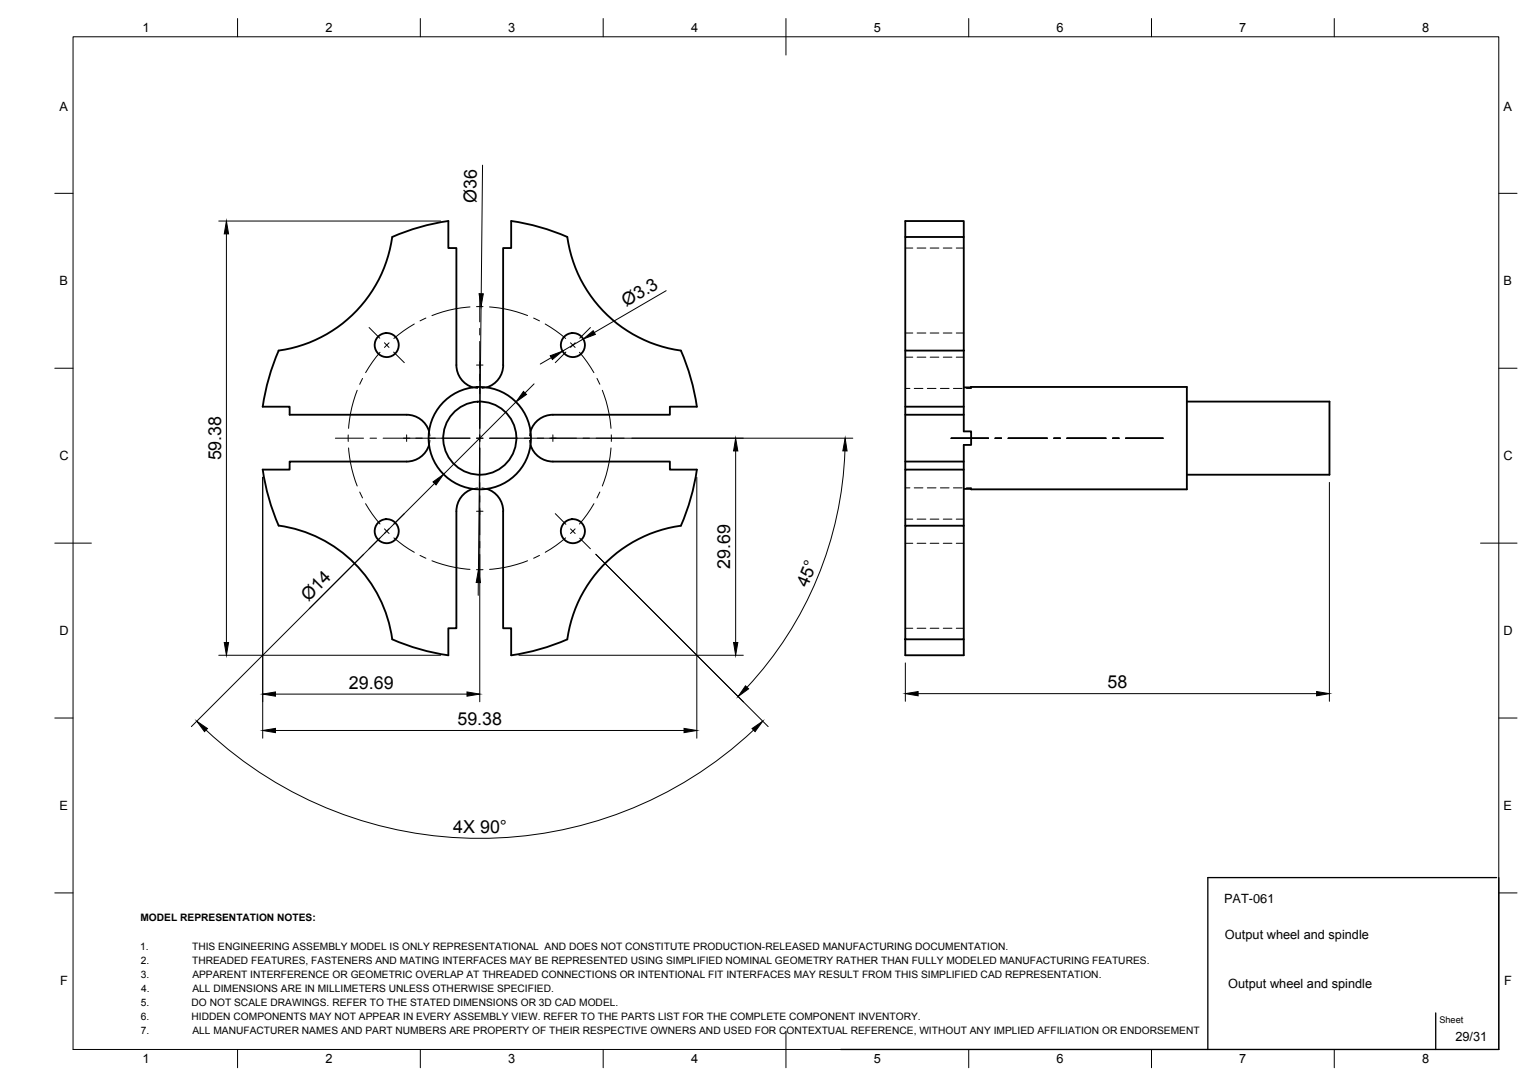
ISO-10303-21;
HEADER;
/* Generated by software containing ST-Developer
 * from STEP Tools, Inc. (www.steptools.com) 
 */

FILE_DESCRIPTION(
/* description */ ('Compact intermittent indexer'),
/* implementation_level */ '2;1');

FILE_NAME(
/* name */ 'Output wheel and spindle.step',
/* time_stamp */ '2026-10-29T16:32:17-07:00',
/* author */ (''),
/* organization */ (''),
/* preprocessor_version */ 'ST-DEVELOPER v20.2',
/* originating_system */ 'Autodesk Translation Framework v15.17.0.0',
/* authorisation */ '');

FILE_SCHEMA (('AUTOMOTIVE_DESIGN { 1 0 10303 214 3 1 1 }'));
ENDSEC;

DATA;
#10=MECHANICAL_DESIGN_GEOMETRIC_PRESENTATION_REPRESENTATION('',(#285),#10837);
#229=SHAPE_REPRESENTATION_RELATIONSHIP('SRR','None',#10966,#253);
#253=ADVANCED_BREP_SHAPE_REPRESENTATION('',(#315),#10833);
#285=STYLED_ITEM('',(#11159),#315);
#315=MANIFOLD_SOLID_BREP('Body1',#5659);
#455=FACE_BOUND('',#1346,.T.);
#456=FACE_BOUND('',#1347,.T.);
#457=FACE_BOUND('',#1348,.T.);
#458=FACE_BOUND('',#1349,.T.);
#459=FACE_BOUND('',#1358,.T.);
#460=FACE_BOUND('',#1360,.T.);
#461=FACE_BOUND('',#1372,.T.);
#462=FACE_BOUND('',#1383,.T.);
#463=FACE_BOUND('',#1397,.T.);
#600=PLANE('',#6521);
#601=PLANE('',#6535);
#602=PLANE('',#6536);
#603=PLANE('',#6537);
#604=PLANE('',#6538);
#605=PLANE('',#6539);
#606=PLANE('',#6540);
#607=PLANE('',#6545);
#608=PLANE('',#6549);
#609=PLANE('',#6561);
#610=PLANE('',#6563);
#611=PLANE('',#6564);
#612=PLANE('',#6565);
#613=PLANE('',#6566);
#614=PLANE('',#6567);
#615=PLANE('',#6568);
#616=PLANE('',#6572);
#617=PLANE('',#6575);
#618=PLANE('',#6577);
#619=PLANE('',#6578);
#620=PLANE('',#6579);
#621=PLANE('',#6580);
#622=PLANE('',#6581);
#623=PLANE('',#6582);
#624=PLANE('',#6586);
#625=PLANE('',#6589);
#626=PLANE('',#6591);
#627=PLANE('',#6592);
#628=PLANE('',#6593);
#629=PLANE('',#6594);
#630=PLANE('',#6595);
#631=PLANE('',#6598);
#632=PLANE('',#6599);
#633=PLANE('',#6600);
#634=PLANE('',#6604);
#904=FACE_OUTER_BOUND('',#1334,.T.);
#905=FACE_OUTER_BOUND('',#1335,.T.);
#906=FACE_OUTER_BOUND('',#1336,.T.);
#907=FACE_OUTER_BOUND('',#1337,.T.);
#908=FACE_OUTER_BOUND('',#1338,.T.);
#909=FACE_OUTER_BOUND('',#1339,.T.);
#910=FACE_OUTER_BOUND('',#1340,.T.);
#911=FACE_OUTER_BOUND('',#1341,.T.);
#912=FACE_OUTER_BOUND('',#1342,.T.);
#913=FACE_OUTER_BOUND('',#1343,.T.);
#914=FACE_OUTER_BOUND('',#1344,.T.);
#915=FACE_OUTER_BOUND('',#1345,.T.);
#916=FACE_OUTER_BOUND('',#1350,.T.);
#917=FACE_OUTER_BOUND('',#1351,.T.);
#918=FACE_OUTER_BOUND('',#1352,.T.);
#919=FACE_OUTER_BOUND('',#1353,.T.);
#920=FACE_OUTER_BOUND('',#1354,.T.);
#921=FACE_OUTER_BOUND('',#1355,.T.);
#922=FACE_OUTER_BOUND('',#1356,.T.);
#923=FACE_OUTER_BOUND('',#1357,.T.);
#924=FACE_OUTER_BOUND('',#1359,.T.);
#925=FACE_OUTER_BOUND('',#1361,.T.);
#926=FACE_OUTER_BOUND('',#1362,.T.);
#927=FACE_OUTER_BOUND('',#1363,.T.);
#928=FACE_OUTER_BOUND('',#1364,.T.);
#929=FACE_OUTER_BOUND('',#1365,.T.);
#930=FACE_OUTER_BOUND('',#1366,.T.);
#931=FACE_OUTER_BOUND('',#1367,.T.);
#932=FACE_OUTER_BOUND('',#1368,.T.);
#933=FACE_OUTER_BOUND('',#1369,.T.);
#934=FACE_OUTER_BOUND('',#1370,.T.);
#935=FACE_OUTER_BOUND('',#1371,.T.);
#936=FACE_OUTER_BOUND('',#1373,.T.);
#937=FACE_OUTER_BOUND('',#1374,.T.);
#938=FACE_OUTER_BOUND('',#1375,.T.);
#939=FACE_OUTER_BOUND('',#1376,.T.);
#940=FACE_OUTER_BOUND('',#1377,.T.);
#941=FACE_OUTER_BOUND('',#1378,.T.);
#942=FACE_OUTER_BOUND('',#1379,.T.);
#943=FACE_OUTER_BOUND('',#1380,.T.);
#944=FACE_OUTER_BOUND('',#1381,.T.);
#945=FACE_OUTER_BOUND('',#1382,.T.);
#946=FACE_OUTER_BOUND('',#1384,.T.);
#947=FACE_OUTER_BOUND('',#1385,.T.);
#948=FACE_OUTER_BOUND('',#1386,.T.);
#949=FACE_OUTER_BOUND('',#1387,.T.);
#950=FACE_OUTER_BOUND('',#1388,.T.);
#951=FACE_OUTER_BOUND('',#1389,.T.);
#952=FACE_OUTER_BOUND('',#1390,.T.);
#953=FACE_OUTER_BOUND('',#1391,.T.);
#954=FACE_OUTER_BOUND('',#1392,.T.);
#955=FACE_OUTER_BOUND('',#1393,.T.);
#956=FACE_OUTER_BOUND('',#1394,.T.);
#957=FACE_OUTER_BOUND('',#1395,.T.);
#958=FACE_OUTER_BOUND('',#1396,.T.);
#959=FACE_OUTER_BOUND('',#1398,.T.);
#960=FACE_OUTER_BOUND('',#1399,.T.);
#1334=EDGE_LOOP('',(#4732,#4733,#4734,#4735));
#1335=EDGE_LOOP('',(#4736,#4737,#4738,#4739));
#1336=EDGE_LOOP('',(#4740,#4741,#4742,#4743));
#1337=EDGE_LOOP('',(#4744,#4745,#4746,#4747));
#1338=EDGE_LOOP('',(#4748,#4749,#4750,#4751));
#1339=EDGE_LOOP('',(#4752,#4753,#4754,#4755));
#1340=EDGE_LOOP('',(#4756,#4757,#4758,#4759));
#1341=EDGE_LOOP('',(#4760,#4761,#4762,#4763));
#1342=EDGE_LOOP('',(#4764,#4765,#4766,#4767));
#1343=EDGE_LOOP('',(#4768,#4769,#4770,#4771));
#1344=EDGE_LOOP('',(#4772,#4773,#4774,#4775));
#1345=EDGE_LOOP('',(#4776,#4777,#4778,#4779,#4780,#4781,#4782,#4783,#4784,
#4785,#4786,#4787,#4788,#4789,#4790,#4791,#4792,#4793,#4794,#4795,#4796,
#4797,#4798,#4799,#4800,#4801,#4802,#4803,#4804,#4805,#4806,#4807,#4808,
#4809,#4810,#4811,#4812,#4813,#4814,#4815));
#1346=EDGE_LOOP('',(#4816));
#1347=EDGE_LOOP('',(#4817));
#1348=EDGE_LOOP('',(#4818));
#1349=EDGE_LOOP('',(#4819));
#1350=EDGE_LOOP('',(#4820,#4821,#4822,#4823));
#1351=EDGE_LOOP('',(#4824,#4825,#4826,#4827));
#1352=EDGE_LOOP('',(#4828,#4829,#4830,#4831));
#1353=EDGE_LOOP('',(#4832,#4833,#4834,#4835));
#1354=EDGE_LOOP('',(#4836,#4837,#4838,#4839));
#1355=EDGE_LOOP('',(#4840,#4841,#4842,#4843));
#1356=EDGE_LOOP('',(#4844,#4845,#4846,#4847));
#1357=EDGE_LOOP('',(#4848,#4849,#4850,#4851,#4852,#4853,#4854,#4855,#4856,
#4857,#4858,#4859));
#1358=EDGE_LOOP('',(#4860));
#1359=EDGE_LOOP('',(#4861,#4862,#4863,#4864,#4865,#4866,#4867,#4868,#4869,
#4870,#4871,#4872));
#1360=EDGE_LOOP('',(#4873));
#1361=EDGE_LOOP('',(#4874,#4875));
#1362=EDGE_LOOP('',(#4876,#4877,#4878,#4879,#4880,#4881,#4882,#4883));
#1363=EDGE_LOOP('',(#4884,#4885,#4886,#4887,#4888,#4889,#4890,#4891,#4892,
#4893,#4894,#4895,#4896,#4897,#4898,#4899,#4900,#4901,#4902,#4903));
#1364=EDGE_LOOP('',(#4904,#4905,#4906,#4907));
#1365=EDGE_LOOP('',(#4908,#4909,#4910,#4911));
#1366=EDGE_LOOP('',(#4912,#4913,#4914,#4915));
#1367=EDGE_LOOP('',(#4916,#4917,#4918,#4919));
#1368=EDGE_LOOP('',(#4920,#4921,#4922,#4923));
#1369=EDGE_LOOP('',(#4924,#4925,#4926,#4927));
#1370=EDGE_LOOP('',(#4928,#4929,#4930,#4931));
#1371=EDGE_LOOP('',(#4932,#4933,#4934,#4935,#4936,#4937,#4938,#4939,#4940,
#4941,#4942,#4943));
#1372=EDGE_LOOP('',(#4944));
#1373=EDGE_LOOP('',(#4945,#4946,#4947));
#1374=EDGE_LOOP('',(#4948,#4949,#4950,#4951,#4952,#4953,#4954,#4955));
#1375=EDGE_LOOP('',(#4956,#4957,#4958,#4959));
#1376=EDGE_LOOP('',(#4960,#4961,#4962,#4963));
#1377=EDGE_LOOP('',(#4964,#4965,#4966,#4967));
#1378=EDGE_LOOP('',(#4968,#4969,#4970,#4971));
#1379=EDGE_LOOP('',(#4972,#4973,#4974,#4975));
#1380=EDGE_LOOP('',(#4976,#4977,#4978,#4979));
#1381=EDGE_LOOP('',(#4980,#4981,#4982,#4983));
#1382=EDGE_LOOP('',(#4984,#4985,#4986,#4987,#4988,#4989,#4990,#4991,#4992,
#4993,#4994,#4995));
#1383=EDGE_LOOP('',(#4996));
#1384=EDGE_LOOP('',(#4997,#4998));
#1385=EDGE_LOOP('',(#4999,#5000,#5001,#5002,#5003,#5004,#5005,#5006));
#1386=EDGE_LOOP('',(#5007,#5008,#5009,#5010));
#1387=EDGE_LOOP('',(#5011,#5012,#5013,#5014));
#1388=EDGE_LOOP('',(#5015,#5016,#5017,#5018));
#1389=EDGE_LOOP('',(#5019,#5020,#5021,#5022));
#1390=EDGE_LOOP('',(#5023,#5024,#5025,#5026));
#1391=EDGE_LOOP('',(#5027,#5028,#5029,#5030));
#1392=EDGE_LOOP('',(#5031,#5032));
#1393=EDGE_LOOP('',(#5033,#5034,#5035,#5036,#5037,#5038,#5039,#5040));
#1394=EDGE_LOOP('',(#5041,#5042,#5043,#5044));
#1395=EDGE_LOOP('',(#5045,#5046,#5047,#5048));
#1396=EDGE_LOOP('',(#5049));
#1397=EDGE_LOOP('',(#5050));
#1398=EDGE_LOOP('',(#5051,#5052,#5053,#5054));
#1399=EDGE_LOOP('',(#5055));
#1656=LINE('',#10192,#2014);
#1657=LINE('',#10198,#2015);
#1658=LINE('',#10204,#2016);
#1659=LINE('',#10210,#2017);
#1660=LINE('',#10217,#2018);
#1661=LINE('',#10220,#2019);
#1662=LINE('',#10226,#2020);
#1663=LINE('',#10229,#2021);
#1664=LINE('',#10235,#2022);
#1665=LINE('',#10238,#2023);
#1666=LINE('',#10242,#2024);
#1667=LINE('',#10246,#2025);
#1668=LINE('',#10252,#2026);
#1669=LINE('',#10258,#2027);
#1670=LINE('',#10264,#2028);
#1671=LINE('',#10268,#2029);
#1672=LINE('',#10270,#2030);
#1673=LINE('',#10272,#2031);
#1674=LINE('',#10276,#2032);
#1675=LINE('',#10278,#2033);
#1676=LINE('',#10280,#2034);
#1677=LINE('',#10285,#2035);
#1678=LINE('',#10287,#2036);
#1679=LINE('',#10289,#2037);
#1680=LINE('',#10293,#2038);
#1681=LINE('',#10295,#2039);
#1682=LINE('',#10297,#2040);
#1683=LINE('',#10300,#2041);
#1684=LINE('',#10302,#2042);
#1685=LINE('',#10304,#2043);
#1686=LINE('',#10308,#2044);
#1687=LINE('',#10310,#2045);
#1688=LINE('',#10312,#2046);
#1689=LINE('',#10315,#2047);
#1690=LINE('',#10317,#2048);
#1691=LINE('',#10319,#2049);
#1692=LINE('',#10323,#2050);
#1693=LINE('',#10325,#2051);
#1694=LINE('',#10327,#2052);
#1695=LINE('',#10332,#2053);
#1696=LINE('',#10335,#2054);
#1697=LINE('',#10339,#2055);
#1698=LINE('',#10340,#2056);
#1699=LINE('',#10343,#2057);
#1700=LINE('',#10344,#2058);
#1701=LINE('',#10347,#2059);
#1702=LINE('',#10349,#2060);
#1703=LINE('',#10350,#2061);
#1704=LINE('',#10352,#2062);
#1705=LINE('',#10355,#2063);
#1706=LINE('',#10356,#2064);
#1707=LINE('',#10361,#2065);
#1708=LINE('',#10363,#2066);
#1709=LINE('',#10365,#2067);
#1710=LINE('',#10373,#2068);
#1711=LINE('',#10381,#2069);
#1712=LINE('',#10383,#2070);
#1713=LINE('',#10384,#2071);
#1714=LINE('',#10391,#2072);
#1715=LINE('',#10392,#2073);
#1716=LINE('',#10393,#2074);
#1717=LINE('',#10396,#2075);
#1718=LINE('',#10400,#2076);
#1719=LINE('',#10405,#2077);
#1720=LINE('',#10409,#2078);
#1721=LINE('',#10413,#2079);
#1722=LINE('',#10417,#2080);
#1723=LINE('',#10420,#2081);
#1724=LINE('',#10423,#2082);
#1725=LINE('',#10425,#2083);
#1726=LINE('',#10427,#2084);
#1727=LINE('',#10430,#2085);
#1728=LINE('',#10432,#2086);
#1729=LINE('',#10433,#2087);
#1730=LINE('',#10435,#2088);
#1731=LINE('',#10438,#2089);
#1732=LINE('',#10439,#2090);
#1733=LINE('',#10444,#2091);
#1734=LINE('',#10446,#2092);
#1735=LINE('',#10448,#2093);
#1736=LINE('',#10454,#2094);
#1737=LINE('',#10457,#2095);
#1738=LINE('',#10459,#2096);
#1739=LINE('',#10461,#2097);
#1740=LINE('',#10464,#2098);
#1741=LINE('',#10466,#2099);
#1742=LINE('',#10467,#2100);
#1743=LINE('',#10469,#2101);
#1744=LINE('',#10472,#2102);
#1745=LINE('',#10473,#2103);
#1746=LINE('',#10478,#2104);
#1747=LINE('',#10480,#2105);
#1748=LINE('',#10482,#2106);
#1749=LINE('',#10488,#2107);
#1750=LINE('',#10491,#2108);
#1751=LINE('',#10493,#2109);
#1752=LINE('',#10495,#2110);
#1753=LINE('',#10497,#2111);
#1754=LINE('',#10499,#2112);
#1755=LINE('',#10503,#2113);
#1756=LINE('',#10504,#2114);
#1757=LINE('',#10512,#2115);
#2014=VECTOR('',#8014,0.165);
#2015=VECTOR('',#8021,0.165);
#2016=VECTOR('',#8028,0.165);
#2017=VECTOR('',#8035,0.165);
#2018=VECTOR('',#8042,1.);
#2019=VECTOR('',#8045,1.);
#2020=VECTOR('',#8050,1.);
#2021=VECTOR('',#8053,1.);
#2022=VECTOR('',#8058,1.);
#2023=VECTOR('',#8061,1.);
#2024=VECTOR('',#8064,1.);
#2025=VECTOR('',#8067,1.);
#2026=VECTOR('',#8074,1.);
#2027=VECTOR('',#8081,1.);
#2028=VECTOR('',#8088,1.);
#2029=VECTOR('',#8093,1.);
#2030=VECTOR('',#8094,1.);
#2031=VECTOR('',#8095,1.);
#2032=VECTOR('',#8098,1.);
#2033=VECTOR('',#8099,1.);
#2034=VECTOR('',#8100,1.);
#2035=VECTOR('',#8105,1.);
#2036=VECTOR('',#8106,1.);
#2037=VECTOR('',#8107,1.);
#2038=VECTOR('',#8110,1.);
#2039=VECTOR('',#8111,1.);
#2040=VECTOR('',#8112,1.);
#2041=VECTOR('',#8115,1.);
#2042=VECTOR('',#8116,1.);
#2043=VECTOR('',#8117,1.);
#2044=VECTOR('',#8120,1.);
#2045=VECTOR('',#8121,1.);
#2046=VECTOR('',#8122,1.);
#2047=VECTOR('',#8125,1.);
#2048=VECTOR('',#8126,1.);
#2049=VECTOR('',#8127,1.);
#2050=VECTOR('',#8130,1.);
#2051=VECTOR('',#8131,1.);
#2052=VECTOR('',#8132,1.);
#2053=VECTOR('',#8139,1.);
#2054=VECTOR('',#8142,1.);
#2055=VECTOR('',#8147,1.);
#2056=VECTOR('',#8148,1.);
#2057=VECTOR('',#8151,1.);
#2058=VECTOR('',#8152,1.);
#2059=VECTOR('',#8155,1.);
#2060=VECTOR('',#8156,1.);
#2061=VECTOR('',#8157,1.);
#2062=VECTOR('',#8160,1.);
#2063=VECTOR('',#8163,1.);
#2064=VECTOR('',#8164,1.);
#2065=VECTOR('',#8169,1.);
#2066=VECTOR('',#8170,1.);
#2067=VECTOR('',#8171,1.);
#2068=VECTOR('',#8180,1.);
#2069=VECTOR('',#8187,1.);
#2070=VECTOR('',#8188,1.);
#2071=VECTOR('',#8189,1.);
#2072=VECTOR('',#8198,1.);
#2073=VECTOR('',#8199,1.);
#2074=VECTOR('',#8200,1.);
#2075=VECTOR('',#8203,1.);
#2076=VECTOR('',#8206,0.7);
#2077=VECTOR('',#8211,1.);
#2078=VECTOR('',#8214,1.);
#2079=VECTOR('',#8217,1.);
#2080=VECTOR('',#8220,1.);
#2081=VECTOR('',#8223,1.);
#2082=VECTOR('',#8228,1.);
#2083=VECTOR('',#8231,1.);
#2084=VECTOR('',#8234,1.);
#2085=VECTOR('',#8237,1.);
#2086=VECTOR('',#8238,1.);
#2087=VECTOR('',#8239,1.);
#2088=VECTOR('',#8242,1.);
#2089=VECTOR('',#8245,1.);
#2090=VECTOR('',#8246,1.);
#2091=VECTOR('',#8251,1.);
#2092=VECTOR('',#8252,1.);
#2093=VECTOR('',#8253,1.);
#2094=VECTOR('',#8264,1.);
#2095=VECTOR('',#8269,1.);
#2096=VECTOR('',#8272,1.);
#2097=VECTOR('',#8275,1.);
#2098=VECTOR('',#8278,1.);
#2099=VECTOR('',#8279,1.);
#2100=VECTOR('',#8280,1.);
#2101=VECTOR('',#8283,1.);
#2102=VECTOR('',#8286,1.);
#2103=VECTOR('',#8287,1.);
#2104=VECTOR('',#8292,1.);
#2105=VECTOR('',#8293,1.);
#2106=VECTOR('',#8294,1.);
#2107=VECTOR('',#8305,1.);
#2108=VECTOR('',#8310,1.);
#2109=VECTOR('',#8313,1.);
#2110=VECTOR('',#8316,1.);
#2111=VECTOR('',#8319,1.);
#2112=VECTOR('',#8322,1.);
#2113=VECTOR('',#8329,1.);
#2114=VECTOR('',#8330,1.);
#2115=VECTOR('',#8341,0.5);
#2406=CIRCLE('',#6489,0.165);
#2407=CIRCLE('',#6490,0.165);
#2408=CIRCLE('',#6492,0.165);
#2409=CIRCLE('',#6493,0.165);
#2410=CIRCLE('',#6495,0.165);
#2411=CIRCLE('',#6496,0.165);
#2412=CIRCLE('',#6498,0.165);
#2413=CIRCLE('',#6499,0.165);
#2414=CIRCLE('',#6501,1.82);
#2415=CIRCLE('',#6502,1.82);
#2416=CIRCLE('',#6504,1.82);
#2417=CIRCLE('',#6505,1.82);
#2418=CIRCLE('',#6507,1.82);
#2419=CIRCLE('',#6508,1.82);
#2420=CIRCLE('',#6510,1.82);
#2421=CIRCLE('',#6511,1.82);
#2422=CIRCLE('',#6513,3.);
#2423=CIRCLE('',#6514,3.);
#2424=CIRCLE('',#6516,3.);
#2425=CIRCLE('',#6517,3.);
#2426=CIRCLE('',#6519,3.);
#2427=CIRCLE('',#6520,3.);
#2428=CIRCLE('',#6522,0.32);
#2429=CIRCLE('',#6523,3.);
#2430=CIRCLE('',#6524,3.);
#2431=CIRCLE('',#6525,0.32);
#2432=CIRCLE('',#6526,3.);
#2433=CIRCLE('',#6527,0.32);
#2434=CIRCLE('',#6528,3.);
#2435=CIRCLE('',#6529,0.32);
#2436=CIRCLE('',#6530,3.);
#2437=CIRCLE('',#6532,3.);
#2438=CIRCLE('',#6534,3.);
#2439=CIRCLE('',#6541,3.);
#2440=CIRCLE('',#6542,0.32);
#2441=CIRCLE('',#6543,0.7);
#2442=CIRCLE('',#6544,0.32);
#2443=CIRCLE('',#6546,0.32);
#2444=CIRCLE('',#6547,0.7);
#2445=CIRCLE('',#6548,0.32);
#2446=CIRCLE('',#6550,0.7);
#2447=CIRCLE('',#6551,0.32);
#2448=CIRCLE('',#6554,0.7);
#2449=CIRCLE('',#6555,0.7);
#2450=CIRCLE('',#6556,0.7);
#2451=CIRCLE('',#6557,0.7);
#2452=CIRCLE('',#6558,0.7);
#2453=CIRCLE('',#6559,0.7);
#2454=CIRCLE('',#6560,0.7);
#2455=CIRCLE('',#6569,3.);
#2456=CIRCLE('',#6570,0.32);
#2457=CIRCLE('',#6571,0.32);
#2458=CIRCLE('',#6573,0.32);
#2459=CIRCLE('',#6583,3.);
#2460=CIRCLE('',#6584,0.32);
#2461=CIRCLE('',#6585,0.32);
#2462=CIRCLE('',#6587,0.32);
#2463=CIRCLE('',#6596,0.32);
#2464=CIRCLE('',#6601,0.5);
#2465=CIRCLE('',#6603,0.5);
#2830=VERTEX_POINT('',#10189);
#2831=VERTEX_POINT('',#10191);
#2832=VERTEX_POINT('',#10195);
#2833=VERTEX_POINT('',#10197);
#2834=VERTEX_POINT('',#10201);
#2835=VERTEX_POINT('',#10203);
#2836=VERTEX_POINT('',#10207);
#2837=VERTEX_POINT('',#10209);
#2838=VERTEX_POINT('',#10213);
#2839=VERTEX_POINT('',#10214);
#2840=VERTEX_POINT('',#10216);
#2841=VERTEX_POINT('',#10218);
#2842=VERTEX_POINT('',#10222);
#2843=VERTEX_POINT('',#10223);
#2844=VERTEX_POINT('',#10225);
#2845=VERTEX_POINT('',#10227);
#2846=VERTEX_POINT('',#10231);
#2847=VERTEX_POINT('',#10232);
#2848=VERTEX_POINT('',#10234);
#2849=VERTEX_POINT('',#10236);
#2850=VERTEX_POINT('',#10240);
#2851=VERTEX_POINT('',#10241);
#2852=VERTEX_POINT('',#10243);
#2853=VERTEX_POINT('',#10245);
#2854=VERTEX_POINT('',#10249);
#2855=VERTEX_POINT('',#10251);
#2856=VERTEX_POINT('',#10255);
#2857=VERTEX_POINT('',#10257);
#2858=VERTEX_POINT('',#10261);
#2859=VERTEX_POINT('',#10263);
#2860=VERTEX_POINT('',#10267);
#2861=VERTEX_POINT('',#10269);
#2862=VERTEX_POINT('',#10271);
#2863=VERTEX_POINT('',#10273);
#2864=VERTEX_POINT('',#10275);
#2865=VERTEX_POINT('',#10277);
#2866=VERTEX_POINT('',#10279);
#2867=VERTEX_POINT('',#10282);
#2868=VERTEX_POINT('',#10284);
#2869=VERTEX_POINT('',#10286);
#2870=VERTEX_POINT('',#10288);
#2871=VERTEX_POINT('',#10290);
#2872=VERTEX_POINT('',#10292);
#2873=VERTEX_POINT('',#10294);
#2874=VERTEX_POINT('',#10296);
#2875=VERTEX_POINT('',#10299);
#2876=VERTEX_POINT('',#10301);
#2877=VERTEX_POINT('',#10303);
#2878=VERTEX_POINT('',#10305);
#2879=VERTEX_POINT('',#10307);
#2880=VERTEX_POINT('',#10309);
#2881=VERTEX_POINT('',#10311);
#2882=VERTEX_POINT('',#10314);
#2883=VERTEX_POINT('',#10316);
#2884=VERTEX_POINT('',#10318);
#2885=VERTEX_POINT('',#10320);
#2886=VERTEX_POINT('',#10322);
#2887=VERTEX_POINT('',#10324);
#2888=VERTEX_POINT('',#10326);
#2889=VERTEX_POINT('',#10330);
#2890=VERTEX_POINT('',#10334);
#2891=VERTEX_POINT('',#10338);
#2892=VERTEX_POINT('',#10342);
#2893=VERTEX_POINT('',#10346);
#2894=VERTEX_POINT('',#10348);
#2895=VERTEX_POINT('',#10354);
#2896=VERTEX_POINT('',#10358);
#2897=VERTEX_POINT('',#10360);
#2898=VERTEX_POINT('',#10362);
#2899=VERTEX_POINT('',#10364);
#2900=VERTEX_POINT('',#10366);
#2901=VERTEX_POINT('',#10368);
#2902=VERTEX_POINT('',#10372);
#2903=VERTEX_POINT('',#10374);
#2904=VERTEX_POINT('',#10376);
#2905=VERTEX_POINT('',#10378);
#2906=VERTEX_POINT('',#10380);
#2907=VERTEX_POINT('',#10382);
#2908=VERTEX_POINT('',#10386);
#2909=VERTEX_POINT('',#10387);
#2910=VERTEX_POINT('',#10395);
#2911=VERTEX_POINT('',#10397);
#2912=VERTEX_POINT('',#10399);
#2913=VERTEX_POINT('',#10402);
#2914=VERTEX_POINT('',#10404);
#2915=VERTEX_POINT('',#10406);
#2916=VERTEX_POINT('',#10408);
#2917=VERTEX_POINT('',#10410);
#2918=VERTEX_POINT('',#10412);
#2919=VERTEX_POINT('',#10414);
#2920=VERTEX_POINT('',#10416);
#2921=VERTEX_POINT('',#10418);
#2922=VERTEX_POINT('',#10429);
#2923=VERTEX_POINT('',#10431);
#2924=VERTEX_POINT('',#10437);
#2925=VERTEX_POINT('',#10441);
#2926=VERTEX_POINT('',#10443);
#2927=VERTEX_POINT('',#10445);
#2928=VERTEX_POINT('',#10447);
#2929=VERTEX_POINT('',#10463);
#2930=VERTEX_POINT('',#10465);
#2931=VERTEX_POINT('',#10471);
#2932=VERTEX_POINT('',#10475);
#2933=VERTEX_POINT('',#10477);
#2934=VERTEX_POINT('',#10479);
#2935=VERTEX_POINT('',#10481);
#2936=VERTEX_POINT('',#10508);
#2937=VERTEX_POINT('',#10511);
#3488=EDGE_CURVE('',#2830,#2830,#2406,.T.);
#3489=EDGE_CURVE('',#2830,#2831,#1656,.T.);
#3490=EDGE_CURVE('',#2831,#2831,#2407,.T.);
#3491=EDGE_CURVE('',#2832,#2832,#2408,.T.);
#3492=EDGE_CURVE('',#2832,#2833,#1657,.T.);
#3493=EDGE_CURVE('',#2833,#2833,#2409,.T.);
#3494=EDGE_CURVE('',#2834,#2834,#2410,.T.);
#3495=EDGE_CURVE('',#2834,#2835,#1658,.T.);
#3496=EDGE_CURVE('',#2835,#2835,#2411,.T.);
#3497=EDGE_CURVE('',#2836,#2836,#2412,.T.);
#3498=EDGE_CURVE('',#2836,#2837,#1659,.T.);
#3499=EDGE_CURVE('',#2837,#2837,#2413,.T.);
#3500=EDGE_CURVE('',#2838,#2839,#2414,.T.);
#3501=EDGE_CURVE('',#2840,#2838,#1660,.T.);
#3502=EDGE_CURVE('',#2841,#2840,#2415,.T.);
#3503=EDGE_CURVE('',#2839,#2841,#1661,.T.);
#3504=EDGE_CURVE('',#2842,#2843,#2416,.T.);
#3505=EDGE_CURVE('',#2844,#2842,#1662,.T.);
#3506=EDGE_CURVE('',#2845,#2844,#2417,.T.);
#3507=EDGE_CURVE('',#2843,#2845,#1663,.T.);
#3508=EDGE_CURVE('',#2846,#2847,#2418,.T.);
#3509=EDGE_CURVE('',#2848,#2846,#1664,.T.);
#3510=EDGE_CURVE('',#2849,#2848,#2419,.T.);
#3511=EDGE_CURVE('',#2847,#2849,#1665,.T.);
#3512=EDGE_CURVE('',#2850,#2851,#1666,.T.);
#3513=EDGE_CURVE('',#2852,#2850,#2420,.T.);
#3514=EDGE_CURVE('',#2853,#2852,#1667,.T.);
#3515=EDGE_CURVE('',#2851,#2853,#2421,.T.);
#3516=EDGE_CURVE('',#2838,#2854,#2422,.T.);
#3517=EDGE_CURVE('',#2854,#2855,#1668,.T.);
#3518=EDGE_CURVE('',#2840,#2855,#2423,.T.);
#3519=EDGE_CURVE('',#2842,#2856,#2424,.T.);
#3520=EDGE_CURVE('',#2856,#2857,#1669,.T.);
#3521=EDGE_CURVE('',#2844,#2857,#2425,.T.);
#3522=EDGE_CURVE('',#2846,#2858,#2426,.T.);
#3523=EDGE_CURVE('',#2858,#2859,#1670,.T.);
#3524=EDGE_CURVE('',#2848,#2859,#2427,.T.);
#3525=EDGE_CURVE('',#2855,#2860,#1671,.T.);
#3526=EDGE_CURVE('',#2860,#2861,#1672,.T.);
#3527=EDGE_CURVE('',#2861,#2862,#1673,.T.);
#3528=EDGE_CURVE('',#2862,#2863,#2428,.T.);
#3529=EDGE_CURVE('',#2863,#2864,#1674,.T.);
#3530=EDGE_CURVE('',#2864,#2865,#1675,.T.);
#3531=EDGE_CURVE('',#2865,#2866,#1676,.T.);
#3532=EDGE_CURVE('',#2866,#2852,#2429,.T.);
#3533=EDGE_CURVE('',#2850,#2867,#2430,.T.);
#3534=EDGE_CURVE('',#2867,#2868,#1677,.T.);
#3535=EDGE_CURVE('',#2868,#2869,#1678,.T.);
#3536=EDGE_CURVE('',#2869,#2870,#1679,.T.);
#3537=EDGE_CURVE('',#2870,#2871,#2431,.T.);
#3538=EDGE_CURVE('',#2871,#2872,#1680,.T.);
#3539=EDGE_CURVE('',#2872,#2873,#1681,.T.);
#3540=EDGE_CURVE('',#2873,#2874,#1682,.T.);
#3541=EDGE_CURVE('',#2874,#2849,#2432,.T.);
#3542=EDGE_CURVE('',#2859,#2875,#1683,.T.);
#3543=EDGE_CURVE('',#2875,#2876,#1684,.T.);
#3544=EDGE_CURVE('',#2876,#2877,#1685,.T.);
#3545=EDGE_CURVE('',#2877,#2878,#2433,.T.);
#3546=EDGE_CURVE('',#2878,#2879,#1686,.T.);
#3547=EDGE_CURVE('',#2879,#2880,#1687,.T.);
#3548=EDGE_CURVE('',#2880,#2881,#1688,.T.);
#3549=EDGE_CURVE('',#2881,#2845,#2434,.T.);
#3550=EDGE_CURVE('',#2857,#2882,#1689,.T.);
#3551=EDGE_CURVE('',#2882,#2883,#1690,.T.);
#3552=EDGE_CURVE('',#2883,#2884,#1691,.T.);
#3553=EDGE_CURVE('',#2884,#2885,#2435,.T.);
#3554=EDGE_CURVE('',#2885,#2886,#1692,.T.);
#3555=EDGE_CURVE('',#2886,#2887,#1693,.T.);
#3556=EDGE_CURVE('',#2887,#2888,#1694,.T.);
#3557=EDGE_CURVE('',#2888,#2841,#2436,.T.);
#3558=EDGE_CURVE('',#2851,#2889,#2437,.T.);
#3559=EDGE_CURVE('',#2889,#2867,#1695,.T.);
#3560=EDGE_CURVE('',#2866,#2890,#1696,.T.);
#3561=EDGE_CURVE('',#2890,#2853,#2438,.T.);
#3562=EDGE_CURVE('',#2891,#2865,#1697,.T.);
#3563=EDGE_CURVE('',#2890,#2891,#1698,.T.);
#3564=EDGE_CURVE('',#2892,#2864,#1699,.T.);
#3565=EDGE_CURVE('',#2891,#2892,#1700,.T.);
#3566=EDGE_CURVE('',#2893,#2860,#1701,.T.);
#3567=EDGE_CURVE('',#2894,#2893,#1702,.T.);
#3568=EDGE_CURVE('',#2861,#2894,#1703,.T.);
#3569=EDGE_CURVE('',#2893,#2854,#1704,.T.);
#3570=EDGE_CURVE('',#2895,#2894,#1705,.T.);
#3571=EDGE_CURVE('',#2895,#2862,#1706,.T.);
#3572=EDGE_CURVE('',#2896,#2839,#2439,.T.);
#3573=EDGE_CURVE('',#2896,#2897,#1707,.T.);
#3574=EDGE_CURVE('',#2897,#2898,#1708,.T.);
#3575=EDGE_CURVE('',#2898,#2899,#1709,.T.);
#3576=EDGE_CURVE('',#2899,#2900,#2440,.T.);
#3577=EDGE_CURVE('',#2900,#2901,#2441,.T.);
#3578=EDGE_CURVE('',#2901,#2895,#2442,.T.);
#3579=EDGE_CURVE('',#2892,#2902,#1710,.T.);
#3580=EDGE_CURVE('',#2902,#2903,#2443,.T.);
#3581=EDGE_CURVE('',#2903,#2904,#2444,.T.);
#3582=EDGE_CURVE('',#2904,#2905,#2445,.T.);
#3583=EDGE_CURVE('',#2905,#2906,#1711,.T.);
#3584=EDGE_CURVE('',#2906,#2907,#1712,.T.);
#3585=EDGE_CURVE('',#2907,#2889,#1713,.T.);
#3586=EDGE_CURVE('',#2908,#2909,#2446,.T.);
#3587=EDGE_CURVE('',#2908,#2909,#2447,.T.);
#3588=EDGE_CURVE('',#2903,#2908,#1714,.T.);
#3589=EDGE_CURVE('',#2902,#2863,#1715,.T.);
#3590=EDGE_CURVE('',#2909,#2901,#1716,.T.);
#3591=EDGE_CURVE('',#2900,#2910,#1717,.T.);
#3592=EDGE_CURVE('',#2910,#2911,#2448,.T.);
#3593=EDGE_CURVE('',#2911,#2912,#1718,.T.);
#3594=EDGE_CURVE('',#2912,#2912,#2449,.T.);
#3595=EDGE_CURVE('',#2911,#2913,#2450,.T.);
#3596=EDGE_CURVE('',#2913,#2914,#1719,.T.);
#3597=EDGE_CURVE('',#2915,#2914,#2451,.T.);
#3598=EDGE_CURVE('',#2915,#2916,#1720,.T.);
#3599=EDGE_CURVE('',#2916,#2917,#2452,.T.);
#3600=EDGE_CURVE('',#2917,#2918,#1721,.T.);
#3601=EDGE_CURVE('',#2919,#2918,#2453,.T.);
#3602=EDGE_CURVE('',#2919,#2920,#1722,.T.);
#3603=EDGE_CURVE('',#2920,#2921,#2454,.T.);
#3604=EDGE_CURVE('',#2921,#2904,#1723,.T.);
#3605=EDGE_CURVE('',#2888,#2896,#1724,.T.);
#3606=EDGE_CURVE('',#2897,#2887,#1725,.T.);
#3607=EDGE_CURVE('',#2898,#2886,#1726,.T.);
#3608=EDGE_CURVE('',#2922,#2882,#1727,.T.);
#3609=EDGE_CURVE('',#2923,#2922,#1728,.T.);
#3610=EDGE_CURVE('',#2883,#2923,#1729,.T.);
#3611=EDGE_CURVE('',#2922,#2856,#1730,.T.);
#3612=EDGE_CURVE('',#2924,#2923,#1731,.T.);
#3613=EDGE_CURVE('',#2924,#2884,#1732,.T.);
#3614=EDGE_CURVE('',#2925,#2843,#2455,.T.);
#3615=EDGE_CURVE('',#2925,#2926,#1733,.T.);
#3616=EDGE_CURVE('',#2926,#2927,#1734,.T.);
#3617=EDGE_CURVE('',#2927,#2928,#1735,.T.);
#3618=EDGE_CURVE('',#2928,#2915,#2456,.T.);
#3619=EDGE_CURVE('',#2914,#2924,#2457,.T.);
#3620=EDGE_CURVE('',#2910,#2913,#2458,.T.);
#3621=EDGE_CURVE('',#2899,#2885,#1736,.T.);
#3622=EDGE_CURVE('',#2881,#2925,#1737,.T.);
#3623=EDGE_CURVE('',#2926,#2880,#1738,.T.);
#3624=EDGE_CURVE('',#2927,#2879,#1739,.T.);
#3625=EDGE_CURVE('',#2929,#2875,#1740,.T.);
#3626=EDGE_CURVE('',#2930,#2929,#1741,.T.);
#3627=EDGE_CURVE('',#2876,#2930,#1742,.T.);
#3628=EDGE_CURVE('',#2929,#2858,#1743,.T.);
#3629=EDGE_CURVE('',#2931,#2930,#1744,.T.);
#3630=EDGE_CURVE('',#2931,#2877,#1745,.T.);
#3631=EDGE_CURVE('',#2932,#2847,#2459,.T.);
#3632=EDGE_CURVE('',#2932,#2933,#1746,.T.);
#3633=EDGE_CURVE('',#2933,#2934,#1747,.T.);
#3634=EDGE_CURVE('',#2934,#2935,#1748,.T.);
#3635=EDGE_CURVE('',#2935,#2919,#2460,.T.);
#3636=EDGE_CURVE('',#2918,#2931,#2461,.T.);
#3637=EDGE_CURVE('',#2916,#2917,#2462,.T.);
#3638=EDGE_CURVE('',#2928,#2878,#1749,.T.);
#3639=EDGE_CURVE('',#2874,#2932,#1750,.T.);
#3640=EDGE_CURVE('',#2933,#2873,#1751,.T.);
#3641=EDGE_CURVE('',#2907,#2868,#1752,.T.);
#3642=EDGE_CURVE('',#2869,#2906,#1753,.T.);
#3643=EDGE_CURVE('',#2934,#2872,#1754,.T.);
#3644=EDGE_CURVE('',#2920,#2921,#2463,.T.);
#3645=EDGE_CURVE('',#2935,#2871,#1755,.T.);
#3646=EDGE_CURVE('',#2905,#2870,#1756,.T.);
#3647=EDGE_CURVE('',#2936,#2936,#2464,.T.);
#3648=EDGE_CURVE('',#2936,#2937,#1757,.T.);
#3649=EDGE_CURVE('',#2937,#2937,#2465,.T.);
#4732=ORIENTED_EDGE('',*,*,#3488,.F.);
#4733=ORIENTED_EDGE('',*,*,#3489,.T.);
#4734=ORIENTED_EDGE('',*,*,#3490,.F.);
#4735=ORIENTED_EDGE('',*,*,#3489,.F.);
#4736=ORIENTED_EDGE('',*,*,#3491,.F.);
#4737=ORIENTED_EDGE('',*,*,#3492,.T.);
#4738=ORIENTED_EDGE('',*,*,#3493,.F.);
#4739=ORIENTED_EDGE('',*,*,#3492,.F.);
#4740=ORIENTED_EDGE('',*,*,#3494,.F.);
#4741=ORIENTED_EDGE('',*,*,#3495,.T.);
#4742=ORIENTED_EDGE('',*,*,#3496,.F.);
#4743=ORIENTED_EDGE('',*,*,#3495,.F.);
#4744=ORIENTED_EDGE('',*,*,#3497,.F.);
#4745=ORIENTED_EDGE('',*,*,#3498,.T.);
#4746=ORIENTED_EDGE('',*,*,#3499,.F.);
#4747=ORIENTED_EDGE('',*,*,#3498,.F.);
#4748=ORIENTED_EDGE('',*,*,#3500,.F.);
#4749=ORIENTED_EDGE('',*,*,#3501,.F.);
#4750=ORIENTED_EDGE('',*,*,#3502,.F.);
#4751=ORIENTED_EDGE('',*,*,#3503,.F.);
#4752=ORIENTED_EDGE('',*,*,#3504,.F.);
#4753=ORIENTED_EDGE('',*,*,#3505,.F.);
#4754=ORIENTED_EDGE('',*,*,#3506,.F.);
#4755=ORIENTED_EDGE('',*,*,#3507,.F.);
#4756=ORIENTED_EDGE('',*,*,#3508,.F.);
#4757=ORIENTED_EDGE('',*,*,#3509,.F.);
#4758=ORIENTED_EDGE('',*,*,#3510,.F.);
#4759=ORIENTED_EDGE('',*,*,#3511,.F.);
#4760=ORIENTED_EDGE('',*,*,#3512,.F.);
#4761=ORIENTED_EDGE('',*,*,#3513,.F.);
#4762=ORIENTED_EDGE('',*,*,#3514,.F.);
#4763=ORIENTED_EDGE('',*,*,#3515,.F.);
#4764=ORIENTED_EDGE('',*,*,#3501,.T.);
#4765=ORIENTED_EDGE('',*,*,#3516,.T.);
#4766=ORIENTED_EDGE('',*,*,#3517,.T.);
#4767=ORIENTED_EDGE('',*,*,#3518,.F.);
#4768=ORIENTED_EDGE('',*,*,#3505,.T.);
#4769=ORIENTED_EDGE('',*,*,#3519,.T.);
#4770=ORIENTED_EDGE('',*,*,#3520,.T.);
#4771=ORIENTED_EDGE('',*,*,#3521,.F.);
#4772=ORIENTED_EDGE('',*,*,#3509,.T.);
#4773=ORIENTED_EDGE('',*,*,#3522,.T.);
#4774=ORIENTED_EDGE('',*,*,#3523,.T.);
#4775=ORIENTED_EDGE('',*,*,#3524,.F.);
#4776=ORIENTED_EDGE('',*,*,#3502,.T.);
#4777=ORIENTED_EDGE('',*,*,#3518,.T.);
#4778=ORIENTED_EDGE('',*,*,#3525,.T.);
#4779=ORIENTED_EDGE('',*,*,#3526,.T.);
#4780=ORIENTED_EDGE('',*,*,#3527,.T.);
#4781=ORIENTED_EDGE('',*,*,#3528,.T.);
#4782=ORIENTED_EDGE('',*,*,#3529,.T.);
#4783=ORIENTED_EDGE('',*,*,#3530,.T.);
#4784=ORIENTED_EDGE('',*,*,#3531,.T.);
#4785=ORIENTED_EDGE('',*,*,#3532,.T.);
#4786=ORIENTED_EDGE('',*,*,#3513,.T.);
#4787=ORIENTED_EDGE('',*,*,#3533,.T.);
#4788=ORIENTED_EDGE('',*,*,#3534,.T.);
#4789=ORIENTED_EDGE('',*,*,#3535,.T.);
#4790=ORIENTED_EDGE('',*,*,#3536,.T.);
#4791=ORIENTED_EDGE('',*,*,#3537,.T.);
#4792=ORIENTED_EDGE('',*,*,#3538,.T.);
#4793=ORIENTED_EDGE('',*,*,#3539,.T.);
#4794=ORIENTED_EDGE('',*,*,#3540,.T.);
#4795=ORIENTED_EDGE('',*,*,#3541,.T.);
#4796=ORIENTED_EDGE('',*,*,#3510,.T.);
#4797=ORIENTED_EDGE('',*,*,#3524,.T.);
#4798=ORIENTED_EDGE('',*,*,#3542,.T.);
#4799=ORIENTED_EDGE('',*,*,#3543,.T.);
#4800=ORIENTED_EDGE('',*,*,#3544,.T.);
#4801=ORIENTED_EDGE('',*,*,#3545,.T.);
#4802=ORIENTED_EDGE('',*,*,#3546,.T.);
#4803=ORIENTED_EDGE('',*,*,#3547,.T.);
#4804=ORIENTED_EDGE('',*,*,#3548,.T.);
#4805=ORIENTED_EDGE('',*,*,#3549,.T.);
#4806=ORIENTED_EDGE('',*,*,#3506,.T.);
#4807=ORIENTED_EDGE('',*,*,#3521,.T.);
#4808=ORIENTED_EDGE('',*,*,#3550,.T.);
#4809=ORIENTED_EDGE('',*,*,#3551,.T.);
#4810=ORIENTED_EDGE('',*,*,#3552,.T.);
#4811=ORIENTED_EDGE('',*,*,#3553,.T.);
#4812=ORIENTED_EDGE('',*,*,#3554,.T.);
#4813=ORIENTED_EDGE('',*,*,#3555,.T.);
#4814=ORIENTED_EDGE('',*,*,#3556,.T.);
#4815=ORIENTED_EDGE('',*,*,#3557,.T.);
#4816=ORIENTED_EDGE('',*,*,#3490,.T.);
#4817=ORIENTED_EDGE('',*,*,#3493,.T.);
#4818=ORIENTED_EDGE('',*,*,#3496,.T.);
#4819=ORIENTED_EDGE('',*,*,#3499,.T.);
#4820=ORIENTED_EDGE('',*,*,#3512,.T.);
#4821=ORIENTED_EDGE('',*,*,#3558,.T.);
#4822=ORIENTED_EDGE('',*,*,#3559,.T.);
#4823=ORIENTED_EDGE('',*,*,#3533,.F.);
#4824=ORIENTED_EDGE('',*,*,#3514,.T.);
#4825=ORIENTED_EDGE('',*,*,#3532,.F.);
#4826=ORIENTED_EDGE('',*,*,#3560,.T.);
#4827=ORIENTED_EDGE('',*,*,#3561,.T.);
#4828=ORIENTED_EDGE('',*,*,#3531,.F.);
#4829=ORIENTED_EDGE('',*,*,#3562,.F.);
#4830=ORIENTED_EDGE('',*,*,#3563,.F.);
#4831=ORIENTED_EDGE('',*,*,#3560,.F.);
#4832=ORIENTED_EDGE('',*,*,#3530,.F.);
#4833=ORIENTED_EDGE('',*,*,#3564,.F.);
#4834=ORIENTED_EDGE('',*,*,#3565,.F.);
#4835=ORIENTED_EDGE('',*,*,#3562,.T.);
#4836=ORIENTED_EDGE('',*,*,#3526,.F.);
#4837=ORIENTED_EDGE('',*,*,#3566,.F.);
#4838=ORIENTED_EDGE('',*,*,#3567,.F.);
#4839=ORIENTED_EDGE('',*,*,#3568,.F.);
#4840=ORIENTED_EDGE('',*,*,#3525,.F.);
#4841=ORIENTED_EDGE('',*,*,#3517,.F.);
#4842=ORIENTED_EDGE('',*,*,#3569,.F.);
#4843=ORIENTED_EDGE('',*,*,#3566,.T.);
#4844=ORIENTED_EDGE('',*,*,#3568,.T.);
#4845=ORIENTED_EDGE('',*,*,#3570,.F.);
#4846=ORIENTED_EDGE('',*,*,#3571,.T.);
#4847=ORIENTED_EDGE('',*,*,#3527,.F.);
#4848=ORIENTED_EDGE('',*,*,#3500,.T.);
#4849=ORIENTED_EDGE('',*,*,#3572,.F.);
#4850=ORIENTED_EDGE('',*,*,#3573,.T.);
#4851=ORIENTED_EDGE('',*,*,#3574,.T.);
#4852=ORIENTED_EDGE('',*,*,#3575,.T.);
#4853=ORIENTED_EDGE('',*,*,#3576,.T.);
#4854=ORIENTED_EDGE('',*,*,#3577,.T.);
#4855=ORIENTED_EDGE('',*,*,#3578,.T.);
#4856=ORIENTED_EDGE('',*,*,#3570,.T.);
#4857=ORIENTED_EDGE('',*,*,#3567,.T.);
#4858=ORIENTED_EDGE('',*,*,#3569,.T.);
#4859=ORIENTED_EDGE('',*,*,#3516,.F.);
#4860=ORIENTED_EDGE('',*,*,#3488,.T.);
#4861=ORIENTED_EDGE('',*,*,#3515,.T.);
#4862=ORIENTED_EDGE('',*,*,#3561,.F.);
#4863=ORIENTED_EDGE('',*,*,#3563,.T.);
#4864=ORIENTED_EDGE('',*,*,#3565,.T.);
#4865=ORIENTED_EDGE('',*,*,#3579,.T.);
#4866=ORIENTED_EDGE('',*,*,#3580,.T.);
#4867=ORIENTED_EDGE('',*,*,#3581,.T.);
#4868=ORIENTED_EDGE('',*,*,#3582,.T.);
#4869=ORIENTED_EDGE('',*,*,#3583,.T.);
#4870=ORIENTED_EDGE('',*,*,#3584,.T.);
#4871=ORIENTED_EDGE('',*,*,#3585,.T.);
#4872=ORIENTED_EDGE('',*,*,#3558,.F.);
#4873=ORIENTED_EDGE('',*,*,#3497,.T.);
#4874=ORIENTED_EDGE('',*,*,#3586,.F.);
#4875=ORIENTED_EDGE('',*,*,#3587,.T.);
#4876=ORIENTED_EDGE('',*,*,#3588,.F.);
#4877=ORIENTED_EDGE('',*,*,#3580,.F.);
#4878=ORIENTED_EDGE('',*,*,#3589,.T.);
#4879=ORIENTED_EDGE('',*,*,#3528,.F.);
#4880=ORIENTED_EDGE('',*,*,#3571,.F.);
#4881=ORIENTED_EDGE('',*,*,#3578,.F.);
#4882=ORIENTED_EDGE('',*,*,#3590,.F.);
#4883=ORIENTED_EDGE('',*,*,#3587,.F.);
#4884=ORIENTED_EDGE('',*,*,#3588,.T.);
#4885=ORIENTED_EDGE('',*,*,#3586,.T.);
#4886=ORIENTED_EDGE('',*,*,#3590,.T.);
#4887=ORIENTED_EDGE('',*,*,#3577,.F.);
#4888=ORIENTED_EDGE('',*,*,#3591,.T.);
#4889=ORIENTED_EDGE('',*,*,#3592,.T.);
#4890=ORIENTED_EDGE('',*,*,#3593,.T.);
#4891=ORIENTED_EDGE('',*,*,#3594,.T.);
#4892=ORIENTED_EDGE('',*,*,#3593,.F.);
#4893=ORIENTED_EDGE('',*,*,#3595,.T.);
#4894=ORIENTED_EDGE('',*,*,#3596,.T.);
#4895=ORIENTED_EDGE('',*,*,#3597,.F.);
#4896=ORIENTED_EDGE('',*,*,#3598,.T.);
#4897=ORIENTED_EDGE('',*,*,#3599,.T.);
#4898=ORIENTED_EDGE('',*,*,#3600,.T.);
#4899=ORIENTED_EDGE('',*,*,#3601,.F.);
#4900=ORIENTED_EDGE('',*,*,#3602,.T.);
#4901=ORIENTED_EDGE('',*,*,#3603,.T.);
#4902=ORIENTED_EDGE('',*,*,#3604,.T.);
#4903=ORIENTED_EDGE('',*,*,#3581,.F.);
#4904=ORIENTED_EDGE('',*,*,#3564,.T.);
#4905=ORIENTED_EDGE('',*,*,#3529,.F.);
#4906=ORIENTED_EDGE('',*,*,#3589,.F.);
#4907=ORIENTED_EDGE('',*,*,#3579,.F.);
#4908=ORIENTED_EDGE('',*,*,#3503,.T.);
#4909=ORIENTED_EDGE('',*,*,#3557,.F.);
#4910=ORIENTED_EDGE('',*,*,#3605,.T.);
#4911=ORIENTED_EDGE('',*,*,#3572,.T.);
#4912=ORIENTED_EDGE('',*,*,#3556,.F.);
#4913=ORIENTED_EDGE('',*,*,#3606,.F.);
#4914=ORIENTED_EDGE('',*,*,#3573,.F.);
#4915=ORIENTED_EDGE('',*,*,#3605,.F.);
#4916=ORIENTED_EDGE('',*,*,#3555,.F.);
#4917=ORIENTED_EDGE('',*,*,#3607,.F.);
#4918=ORIENTED_EDGE('',*,*,#3574,.F.);
#4919=ORIENTED_EDGE('',*,*,#3606,.T.);
#4920=ORIENTED_EDGE('',*,*,#3551,.F.);
#4921=ORIENTED_EDGE('',*,*,#3608,.F.);
#4922=ORIENTED_EDGE('',*,*,#3609,.F.);
#4923=ORIENTED_EDGE('',*,*,#3610,.F.);
#4924=ORIENTED_EDGE('',*,*,#3550,.F.);
#4925=ORIENTED_EDGE('',*,*,#3520,.F.);
#4926=ORIENTED_EDGE('',*,*,#3611,.F.);
#4927=ORIENTED_EDGE('',*,*,#3608,.T.);
#4928=ORIENTED_EDGE('',*,*,#3610,.T.);
#4929=ORIENTED_EDGE('',*,*,#3612,.F.);
#4930=ORIENTED_EDGE('',*,*,#3613,.T.);
#4931=ORIENTED_EDGE('',*,*,#3552,.F.);
#4932=ORIENTED_EDGE('',*,*,#3504,.T.);
#4933=ORIENTED_EDGE('',*,*,#3614,.F.);
#4934=ORIENTED_EDGE('',*,*,#3615,.T.);
#4935=ORIENTED_EDGE('',*,*,#3616,.T.);
#4936=ORIENTED_EDGE('',*,*,#3617,.T.);
#4937=ORIENTED_EDGE('',*,*,#3618,.T.);
#4938=ORIENTED_EDGE('',*,*,#3597,.T.);
#4939=ORIENTED_EDGE('',*,*,#3619,.T.);
#4940=ORIENTED_EDGE('',*,*,#3612,.T.);
#4941=ORIENTED_EDGE('',*,*,#3609,.T.);
#4942=ORIENTED_EDGE('',*,*,#3611,.T.);
#4943=ORIENTED_EDGE('',*,*,#3519,.F.);
#4944=ORIENTED_EDGE('',*,*,#3491,.T.);
#4945=ORIENTED_EDGE('',*,*,#3592,.F.);
#4946=ORIENTED_EDGE('',*,*,#3620,.T.);
#4947=ORIENTED_EDGE('',*,*,#3595,.F.);
#4948=ORIENTED_EDGE('',*,*,#3591,.F.);
#4949=ORIENTED_EDGE('',*,*,#3576,.F.);
#4950=ORIENTED_EDGE('',*,*,#3621,.T.);
#4951=ORIENTED_EDGE('',*,*,#3553,.F.);
#4952=ORIENTED_EDGE('',*,*,#3613,.F.);
#4953=ORIENTED_EDGE('',*,*,#3619,.F.);
#4954=ORIENTED_EDGE('',*,*,#3596,.F.);
#4955=ORIENTED_EDGE('',*,*,#3620,.F.);
#4956=ORIENTED_EDGE('',*,*,#3607,.T.);
#4957=ORIENTED_EDGE('',*,*,#3554,.F.);
#4958=ORIENTED_EDGE('',*,*,#3621,.F.);
#4959=ORIENTED_EDGE('',*,*,#3575,.F.);
#4960=ORIENTED_EDGE('',*,*,#3507,.T.);
#4961=ORIENTED_EDGE('',*,*,#3549,.F.);
#4962=ORIENTED_EDGE('',*,*,#3622,.T.);
#4963=ORIENTED_EDGE('',*,*,#3614,.T.);
#4964=ORIENTED_EDGE('',*,*,#3548,.F.);
#4965=ORIENTED_EDGE('',*,*,#3623,.F.);
#4966=ORIENTED_EDGE('',*,*,#3615,.F.);
#4967=ORIENTED_EDGE('',*,*,#3622,.F.);
#4968=ORIENTED_EDGE('',*,*,#3547,.F.);
#4969=ORIENTED_EDGE('',*,*,#3624,.F.);
#4970=ORIENTED_EDGE('',*,*,#3616,.F.);
#4971=ORIENTED_EDGE('',*,*,#3623,.T.);
#4972=ORIENTED_EDGE('',*,*,#3543,.F.);
#4973=ORIENTED_EDGE('',*,*,#3625,.F.);
#4974=ORIENTED_EDGE('',*,*,#3626,.F.);
#4975=ORIENTED_EDGE('',*,*,#3627,.F.);
#4976=ORIENTED_EDGE('',*,*,#3542,.F.);
#4977=ORIENTED_EDGE('',*,*,#3523,.F.);
#4978=ORIENTED_EDGE('',*,*,#3628,.F.);
#4979=ORIENTED_EDGE('',*,*,#3625,.T.);
#4980=ORIENTED_EDGE('',*,*,#3627,.T.);
#4981=ORIENTED_EDGE('',*,*,#3629,.F.);
#4982=ORIENTED_EDGE('',*,*,#3630,.T.);
#4983=ORIENTED_EDGE('',*,*,#3544,.F.);
#4984=ORIENTED_EDGE('',*,*,#3508,.T.);
#4985=ORIENTED_EDGE('',*,*,#3631,.F.);
#4986=ORIENTED_EDGE('',*,*,#3632,.T.);
#4987=ORIENTED_EDGE('',*,*,#3633,.T.);
#4988=ORIENTED_EDGE('',*,*,#3634,.T.);
#4989=ORIENTED_EDGE('',*,*,#3635,.T.);
#4990=ORIENTED_EDGE('',*,*,#3601,.T.);
#4991=ORIENTED_EDGE('',*,*,#3636,.T.);
#4992=ORIENTED_EDGE('',*,*,#3629,.T.);
#4993=ORIENTED_EDGE('',*,*,#3626,.T.);
#4994=ORIENTED_EDGE('',*,*,#3628,.T.);
#4995=ORIENTED_EDGE('',*,*,#3522,.F.);
#4996=ORIENTED_EDGE('',*,*,#3494,.T.);
#4997=ORIENTED_EDGE('',*,*,#3599,.F.);
#4998=ORIENTED_EDGE('',*,*,#3637,.T.);
#4999=ORIENTED_EDGE('',*,*,#3598,.F.);
#5000=ORIENTED_EDGE('',*,*,#3618,.F.);
#5001=ORIENTED_EDGE('',*,*,#3638,.T.);
#5002=ORIENTED_EDGE('',*,*,#3545,.F.);
#5003=ORIENTED_EDGE('',*,*,#3630,.F.);
#5004=ORIENTED_EDGE('',*,*,#3636,.F.);
#5005=ORIENTED_EDGE('',*,*,#3600,.F.);
#5006=ORIENTED_EDGE('',*,*,#3637,.F.);
#5007=ORIENTED_EDGE('',*,*,#3624,.T.);
#5008=ORIENTED_EDGE('',*,*,#3546,.F.);
#5009=ORIENTED_EDGE('',*,*,#3638,.F.);
#5010=ORIENTED_EDGE('',*,*,#3617,.F.);
#5011=ORIENTED_EDGE('',*,*,#3511,.T.);
#5012=ORIENTED_EDGE('',*,*,#3541,.F.);
#5013=ORIENTED_EDGE('',*,*,#3639,.T.);
#5014=ORIENTED_EDGE('',*,*,#3631,.T.);
#5015=ORIENTED_EDGE('',*,*,#3540,.F.);
#5016=ORIENTED_EDGE('',*,*,#3640,.F.);
#5017=ORIENTED_EDGE('',*,*,#3632,.F.);
#5018=ORIENTED_EDGE('',*,*,#3639,.F.);
#5019=ORIENTED_EDGE('',*,*,#3585,.F.);
#5020=ORIENTED_EDGE('',*,*,#3641,.T.);
#5021=ORIENTED_EDGE('',*,*,#3534,.F.);
#5022=ORIENTED_EDGE('',*,*,#3559,.F.);
#5023=ORIENTED_EDGE('',*,*,#3584,.F.);
#5024=ORIENTED_EDGE('',*,*,#3642,.F.);
#5025=ORIENTED_EDGE('',*,*,#3535,.F.);
#5026=ORIENTED_EDGE('',*,*,#3641,.F.);
#5027=ORIENTED_EDGE('',*,*,#3539,.F.);
#5028=ORIENTED_EDGE('',*,*,#3643,.F.);
#5029=ORIENTED_EDGE('',*,*,#3633,.F.);
#5030=ORIENTED_EDGE('',*,*,#3640,.T.);
#5031=ORIENTED_EDGE('',*,*,#3603,.F.);
#5032=ORIENTED_EDGE('',*,*,#3644,.T.);
#5033=ORIENTED_EDGE('',*,*,#3602,.F.);
#5034=ORIENTED_EDGE('',*,*,#3635,.F.);
#5035=ORIENTED_EDGE('',*,*,#3645,.T.);
#5036=ORIENTED_EDGE('',*,*,#3537,.F.);
#5037=ORIENTED_EDGE('',*,*,#3646,.F.);
#5038=ORIENTED_EDGE('',*,*,#3582,.F.);
#5039=ORIENTED_EDGE('',*,*,#3604,.F.);
#5040=ORIENTED_EDGE('',*,*,#3644,.F.);
#5041=ORIENTED_EDGE('',*,*,#3643,.T.);
#5042=ORIENTED_EDGE('',*,*,#3538,.F.);
#5043=ORIENTED_EDGE('',*,*,#3645,.F.);
#5044=ORIENTED_EDGE('',*,*,#3634,.F.);
#5045=ORIENTED_EDGE('',*,*,#3642,.T.);
#5046=ORIENTED_EDGE('',*,*,#3583,.F.);
#5047=ORIENTED_EDGE('',*,*,#3646,.T.);
#5048=ORIENTED_EDGE('',*,*,#3536,.F.);
#5049=ORIENTED_EDGE('',*,*,#3594,.F.);
#5050=ORIENTED_EDGE('',*,*,#3647,.F.);
#5051=ORIENTED_EDGE('',*,*,#3647,.T.);
#5052=ORIENTED_EDGE('',*,*,#3648,.T.);
#5053=ORIENTED_EDGE('',*,*,#3649,.T.);
#5054=ORIENTED_EDGE('',*,*,#3648,.F.);
#5055=ORIENTED_EDGE('',*,*,#3649,.F.);
#5266=CYLINDRICAL_SURFACE('',#6488,0.165);
#5267=CYLINDRICAL_SURFACE('',#6491,0.165);
#5268=CYLINDRICAL_SURFACE('',#6494,0.165);
#5269=CYLINDRICAL_SURFACE('',#6497,0.165);
#5270=CYLINDRICAL_SURFACE('',#6500,1.82);
#5271=CYLINDRICAL_SURFACE('',#6503,1.82);
#5272=CYLINDRICAL_SURFACE('',#6506,1.82);
#5273=CYLINDRICAL_SURFACE('',#6509,1.82);
#5274=CYLINDRICAL_SURFACE('',#6512,3.);
#5275=CYLINDRICAL_SURFACE('',#6515,3.);
#5276=CYLINDRICAL_SURFACE('',#6518,3.);
#5277=CYLINDRICAL_SURFACE('',#6531,3.);
#5278=CYLINDRICAL_SURFACE('',#6533,3.);
#5279=CYLINDRICAL_SURFACE('',#6552,0.32);
#5280=CYLINDRICAL_SURFACE('',#6553,0.7);
#5281=CYLINDRICAL_SURFACE('',#6562,3.);
#5282=CYLINDRICAL_SURFACE('',#6574,0.32);
#5283=CYLINDRICAL_SURFACE('',#6576,3.);
#5284=CYLINDRICAL_SURFACE('',#6588,0.32);
#5285=CYLINDRICAL_SURFACE('',#6590,3.);
#5286=CYLINDRICAL_SURFACE('',#6597,0.32);
#5287=CYLINDRICAL_SURFACE('',#6602,0.5);
#5547=ADVANCED_FACE('',(#904),#5266,.F.);
#5548=ADVANCED_FACE('',(#905),#5267,.F.);
#5549=ADVANCED_FACE('',(#906),#5268,.F.);
#5550=ADVANCED_FACE('',(#907),#5269,.F.);
#5551=ADVANCED_FACE('',(#908),#5270,.F.);
#5552=ADVANCED_FACE('',(#909),#5271,.F.);
#5553=ADVANCED_FACE('',(#910),#5272,.F.);
#5554=ADVANCED_FACE('',(#911),#5273,.F.);
#5555=ADVANCED_FACE('',(#912),#5274,.T.);
#5556=ADVANCED_FACE('',(#913),#5275,.T.);
#5557=ADVANCED_FACE('',(#914),#5276,.T.);
#5558=ADVANCED_FACE('',(#915,#455,#456,#457,#458),#600,.T.);
#5559=ADVANCED_FACE('',(#916),#5277,.T.);
#5560=ADVANCED_FACE('',(#917),#5278,.T.);
#5561=ADVANCED_FACE('',(#918),#601,.F.);
#5562=ADVANCED_FACE('',(#919),#602,.F.);
#5563=ADVANCED_FACE('',(#920),#603,.F.);
#5564=ADVANCED_FACE('',(#921),#604,.F.);
#5565=ADVANCED_FACE('',(#922),#605,.F.);
#5566=ADVANCED_FACE('',(#923,#459),#606,.F.);
#5567=ADVANCED_FACE('',(#924,#460),#607,.F.);
#5568=ADVANCED_FACE('',(#925),#608,.T.);
#5569=ADVANCED_FACE('',(#926),#5279,.F.);
#5570=ADVANCED_FACE('',(#927),#5280,.T.);
#5571=ADVANCED_FACE('',(#928),#609,.F.);
#5572=ADVANCED_FACE('',(#929),#5281,.T.);
#5573=ADVANCED_FACE('',(#930),#610,.F.);
#5574=ADVANCED_FACE('',(#931),#611,.F.);
#5575=ADVANCED_FACE('',(#932),#612,.F.);
#5576=ADVANCED_FACE('',(#933),#613,.F.);
#5577=ADVANCED_FACE('',(#934),#614,.F.);
#5578=ADVANCED_FACE('',(#935,#461),#615,.F.);
#5579=ADVANCED_FACE('',(#936),#616,.T.);
#5580=ADVANCED_FACE('',(#937),#5282,.F.);
#5581=ADVANCED_FACE('',(#938),#617,.F.);
#5582=ADVANCED_FACE('',(#939),#5283,.T.);
#5583=ADVANCED_FACE('',(#940),#618,.F.);
#5584=ADVANCED_FACE('',(#941),#619,.F.);
#5585=ADVANCED_FACE('',(#942),#620,.F.);
#5586=ADVANCED_FACE('',(#943),#621,.F.);
#5587=ADVANCED_FACE('',(#944),#622,.F.);
#5588=ADVANCED_FACE('',(#945,#462),#623,.F.);
#5589=ADVANCED_FACE('',(#946),#624,.T.);
#5590=ADVANCED_FACE('',(#947),#5284,.F.);
#5591=ADVANCED_FACE('',(#948),#625,.F.);
#5592=ADVANCED_FACE('',(#949),#5285,.T.);
#5593=ADVANCED_FACE('',(#950),#626,.F.);
#5594=ADVANCED_FACE('',(#951),#627,.F.);
#5595=ADVANCED_FACE('',(#952),#628,.F.);
#5596=ADVANCED_FACE('',(#953),#629,.F.);
#5597=ADVANCED_FACE('',(#954),#630,.T.);
#5598=ADVANCED_FACE('',(#955),#5286,.F.);
#5599=ADVANCED_FACE('',(#956),#631,.F.);
#5600=ADVANCED_FACE('',(#957),#632,.F.);
#5601=ADVANCED_FACE('',(#958,#463),#633,.F.);
#5602=ADVANCED_FACE('',(#959),#5287,.T.);
#5603=ADVANCED_FACE('',(#960),#634,.F.);
#5659=CLOSED_SHELL('',(#5547,#5548,#5549,#5550,#5551,#5552,#5553,#5554,
#5555,#5556,#5557,#5558,#5559,#5560,#5561,#5562,#5563,#5564,#5565,#5566,
#5567,#5568,#5569,#5570,#5571,#5572,#5573,#5574,#5575,#5576,#5577,#5578,
#5579,#5580,#5581,#5582,#5583,#5584,#5585,#5586,#5587,#5588,#5589,#5590,
#5591,#5592,#5593,#5594,#5595,#5596,#5597,#5598,#5599,#5600,#5601,#5602,
#5603));
#6487=AXIS2_PLACEMENT_3D('',#10187,#8008,#8009);
#6488=AXIS2_PLACEMENT_3D('',#10188,#8010,#8011);
#6489=AXIS2_PLACEMENT_3D('',#10190,#8012,#8013);
#6490=AXIS2_PLACEMENT_3D('',#10193,#8015,#8016);
#6491=AXIS2_PLACEMENT_3D('',#10194,#8017,#8018);
#6492=AXIS2_PLACEMENT_3D('',#10196,#8019,#8020);
#6493=AXIS2_PLACEMENT_3D('',#10199,#8022,#8023);
#6494=AXIS2_PLACEMENT_3D('',#10200,#8024,#8025);
#6495=AXIS2_PLACEMENT_3D('',#10202,#8026,#8027);
#6496=AXIS2_PLACEMENT_3D('',#10205,#8029,#8030);
#6497=AXIS2_PLACEMENT_3D('',#10206,#8031,#8032);
#6498=AXIS2_PLACEMENT_3D('',#10208,#8033,#8034);
#6499=AXIS2_PLACEMENT_3D('',#10211,#8036,#8037);
#6500=AXIS2_PLACEMENT_3D('',#10212,#8038,#8039);
#6501=AXIS2_PLACEMENT_3D('',#10215,#8040,#8041);
#6502=AXIS2_PLACEMENT_3D('',#10219,#8043,#8044);
#6503=AXIS2_PLACEMENT_3D('',#10221,#8046,#8047);
#6504=AXIS2_PLACEMENT_3D('',#10224,#8048,#8049);
#6505=AXIS2_PLACEMENT_3D('',#10228,#8051,#8052);
#6506=AXIS2_PLACEMENT_3D('',#10230,#8054,#8055);
#6507=AXIS2_PLACEMENT_3D('',#10233,#8056,#8057);
#6508=AXIS2_PLACEMENT_3D('',#10237,#8059,#8060);
#6509=AXIS2_PLACEMENT_3D('',#10239,#8062,#8063);
#6510=AXIS2_PLACEMENT_3D('',#10244,#8065,#8066);
#6511=AXIS2_PLACEMENT_3D('',#10247,#8068,#8069);
#6512=AXIS2_PLACEMENT_3D('',#10248,#8070,#8071);
#6513=AXIS2_PLACEMENT_3D('',#10250,#8072,#8073);
#6514=AXIS2_PLACEMENT_3D('',#10253,#8075,#8076);
#6515=AXIS2_PLACEMENT_3D('',#10254,#8077,#8078);
#6516=AXIS2_PLACEMENT_3D('',#10256,#8079,#8080);
#6517=AXIS2_PLACEMENT_3D('',#10259,#8082,#8083);
#6518=AXIS2_PLACEMENT_3D('',#10260,#8084,#8085);
#6519=AXIS2_PLACEMENT_3D('',#10262,#8086,#8087);
#6520=AXIS2_PLACEMENT_3D('',#10265,#8089,#8090);
#6521=AXIS2_PLACEMENT_3D('',#10266,#8091,#8092);
#6522=AXIS2_PLACEMENT_3D('',#10274,#8096,#8097);
#6523=AXIS2_PLACEMENT_3D('',#10281,#8101,#8102);
#6524=AXIS2_PLACEMENT_3D('',#10283,#8103,#8104);
#6525=AXIS2_PLACEMENT_3D('',#10291,#8108,#8109);
#6526=AXIS2_PLACEMENT_3D('',#10298,#8113,#8114);
#6527=AXIS2_PLACEMENT_3D('',#10306,#8118,#8119);
#6528=AXIS2_PLACEMENT_3D('',#10313,#8123,#8124);
#6529=AXIS2_PLACEMENT_3D('',#10321,#8128,#8129);
#6530=AXIS2_PLACEMENT_3D('',#10328,#8133,#8134);
#6531=AXIS2_PLACEMENT_3D('',#10329,#8135,#8136);
#6532=AXIS2_PLACEMENT_3D('',#10331,#8137,#8138);
#6533=AXIS2_PLACEMENT_3D('',#10333,#8140,#8141);
#6534=AXIS2_PLACEMENT_3D('',#10336,#8143,#8144);
#6535=AXIS2_PLACEMENT_3D('',#10337,#8145,#8146);
#6536=AXIS2_PLACEMENT_3D('',#10341,#8149,#8150);
#6537=AXIS2_PLACEMENT_3D('',#10345,#8153,#8154);
#6538=AXIS2_PLACEMENT_3D('',#10351,#8158,#8159);
#6539=AXIS2_PLACEMENT_3D('',#10353,#8161,#8162);
#6540=AXIS2_PLACEMENT_3D('',#10357,#8165,#8166);
#6541=AXIS2_PLACEMENT_3D('',#10359,#8167,#8168);
#6542=AXIS2_PLACEMENT_3D('',#10367,#8172,#8173);
#6543=AXIS2_PLACEMENT_3D('',#10369,#8174,#8175);
#6544=AXIS2_PLACEMENT_3D('',#10370,#8176,#8177);
#6545=AXIS2_PLACEMENT_3D('',#10371,#8178,#8179);
#6546=AXIS2_PLACEMENT_3D('',#10375,#8181,#8182);
#6547=AXIS2_PLACEMENT_3D('',#10377,#8183,#8184);
#6548=AXIS2_PLACEMENT_3D('',#10379,#8185,#8186);
#6549=AXIS2_PLACEMENT_3D('',#10385,#8190,#8191);
#6550=AXIS2_PLACEMENT_3D('',#10388,#8192,#8193);
#6551=AXIS2_PLACEMENT_3D('',#10389,#8194,#8195);
#6552=AXIS2_PLACEMENT_3D('',#10390,#8196,#8197);
#6553=AXIS2_PLACEMENT_3D('',#10394,#8201,#8202);
#6554=AXIS2_PLACEMENT_3D('',#10398,#8204,#8205);
#6555=AXIS2_PLACEMENT_3D('',#10401,#8207,#8208);
#6556=AXIS2_PLACEMENT_3D('',#10403,#8209,#8210);
#6557=AXIS2_PLACEMENT_3D('',#10407,#8212,#8213);
#6558=AXIS2_PLACEMENT_3D('',#10411,#8215,#8216);
#6559=AXIS2_PLACEMENT_3D('',#10415,#8218,#8219);
#6560=AXIS2_PLACEMENT_3D('',#10419,#8221,#8222);
#6561=AXIS2_PLACEMENT_3D('',#10421,#8224,#8225);
#6562=AXIS2_PLACEMENT_3D('',#10422,#8226,#8227);
#6563=AXIS2_PLACEMENT_3D('',#10424,#8229,#8230);
#6564=AXIS2_PLACEMENT_3D('',#10426,#8232,#8233);
#6565=AXIS2_PLACEMENT_3D('',#10428,#8235,#8236);
#6566=AXIS2_PLACEMENT_3D('',#10434,#8240,#8241);
#6567=AXIS2_PLACEMENT_3D('',#10436,#8243,#8244);
#6568=AXIS2_PLACEMENT_3D('',#10440,#8247,#8248);
#6569=AXIS2_PLACEMENT_3D('',#10442,#8249,#8250);
#6570=AXIS2_PLACEMENT_3D('',#10449,#8254,#8255);
#6571=AXIS2_PLACEMENT_3D('',#10450,#8256,#8257);
#6572=AXIS2_PLACEMENT_3D('',#10451,#8258,#8259);
#6573=AXIS2_PLACEMENT_3D('',#10452,#8260,#8261);
#6574=AXIS2_PLACEMENT_3D('',#10453,#8262,#8263);
#6575=AXIS2_PLACEMENT_3D('',#10455,#8265,#8266);
#6576=AXIS2_PLACEMENT_3D('',#10456,#8267,#8268);
#6577=AXIS2_PLACEMENT_3D('',#10458,#8270,#8271);
#6578=AXIS2_PLACEMENT_3D('',#10460,#8273,#8274);
#6579=AXIS2_PLACEMENT_3D('',#10462,#8276,#8277);
#6580=AXIS2_PLACEMENT_3D('',#10468,#8281,#8282);
#6581=AXIS2_PLACEMENT_3D('',#10470,#8284,#8285);
#6582=AXIS2_PLACEMENT_3D('',#10474,#8288,#8289);
#6583=AXIS2_PLACEMENT_3D('',#10476,#8290,#8291);
#6584=AXIS2_PLACEMENT_3D('',#10483,#8295,#8296);
#6585=AXIS2_PLACEMENT_3D('',#10484,#8297,#8298);
#6586=AXIS2_PLACEMENT_3D('',#10485,#8299,#8300);
#6587=AXIS2_PLACEMENT_3D('',#10486,#8301,#8302);
#6588=AXIS2_PLACEMENT_3D('',#10487,#8303,#8304);
#6589=AXIS2_PLACEMENT_3D('',#10489,#8306,#8307);
#6590=AXIS2_PLACEMENT_3D('',#10490,#8308,#8309);
#6591=AXIS2_PLACEMENT_3D('',#10492,#8311,#8312);
#6592=AXIS2_PLACEMENT_3D('',#10494,#8314,#8315);
#6593=AXIS2_PLACEMENT_3D('',#10496,#8317,#8318);
#6594=AXIS2_PLACEMENT_3D('',#10498,#8320,#8321);
#6595=AXIS2_PLACEMENT_3D('',#10500,#8323,#8324);
#6596=AXIS2_PLACEMENT_3D('',#10501,#8325,#8326);
#6597=AXIS2_PLACEMENT_3D('',#10502,#8327,#8328);
#6598=AXIS2_PLACEMENT_3D('',#10505,#8331,#8332);
#6599=AXIS2_PLACEMENT_3D('',#10506,#8333,#8334);
#6600=AXIS2_PLACEMENT_3D('',#10507,#8335,#8336);
#6601=AXIS2_PLACEMENT_3D('',#10509,#8337,#8338);
#6602=AXIS2_PLACEMENT_3D('',#10510,#8339,#8340);
#6603=AXIS2_PLACEMENT_3D('',#10513,#8342,#8343);
#6604=AXIS2_PLACEMENT_3D('',#10514,#8344,#8345);
#8008=DIRECTION('axis',(0.,0.,1.));
#8009=DIRECTION('refdir',(1.,0.,0.));
#8010=DIRECTION('center_axis',(0.,0.,1.));
#8011=DIRECTION('ref_axis',(1.,0.,0.));
#8012=DIRECTION('center_axis',(0.,0.,1.));
#8013=DIRECTION('ref_axis',(1.,0.,0.));
#8014=DIRECTION('',(0.,0.,1.));
#8015=DIRECTION('center_axis',(0.,0.,-1.));
#8016=DIRECTION('ref_axis',(1.,0.,0.));
#8017=DIRECTION('center_axis',(0.,0.,1.));
#8018=DIRECTION('ref_axis',(1.,0.,0.));
#8019=DIRECTION('center_axis',(0.,0.,1.));
#8020=DIRECTION('ref_axis',(1.,0.,0.));
#8021=DIRECTION('',(0.,0.,1.));
#8022=DIRECTION('center_axis',(0.,0.,-1.));
#8023=DIRECTION('ref_axis',(1.,0.,0.));
#8024=DIRECTION('center_axis',(0.,0.,1.));
#8025=DIRECTION('ref_axis',(1.,0.,0.));
#8026=DIRECTION('center_axis',(0.,0.,1.));
#8027=DIRECTION('ref_axis',(1.,0.,0.));
#8028=DIRECTION('',(0.,0.,1.));
#8029=DIRECTION('center_axis',(0.,0.,-1.));
#8030=DIRECTION('ref_axis',(1.,0.,0.));
#8031=DIRECTION('center_axis',(0.,0.,1.));
#8032=DIRECTION('ref_axis',(1.,0.,0.));
#8033=DIRECTION('center_axis',(0.,0.,1.));
#8034=DIRECTION('ref_axis',(1.,0.,0.));
#8035=DIRECTION('',(0.,0.,1.));
#8036=DIRECTION('center_axis',(0.,0.,-1.));
#8037=DIRECTION('ref_axis',(1.,0.,0.));
#8038=DIRECTION('center_axis',(0.,0.,1.));
#8039=DIRECTION('ref_axis',(1.,0.,0.));
#8040=DIRECTION('center_axis',(0.,0.,1.));
#8041=DIRECTION('ref_axis',(1.,0.,0.));
#8042=DIRECTION('',(0.,0.,-1.));
#8043=DIRECTION('center_axis',(0.,0.,-1.));
#8044=DIRECTION('ref_axis',(1.,0.,0.));
#8045=DIRECTION('',(0.,0.,1.));
#8046=DIRECTION('center_axis',(0.,0.,1.));
#8047=DIRECTION('ref_axis',(1.,0.,0.));
#8048=DIRECTION('center_axis',(0.,0.,1.));
#8049=DIRECTION('ref_axis',(1.,0.,0.));
#8050=DIRECTION('',(0.,0.,-1.));
#8051=DIRECTION('center_axis',(0.,0.,-1.));
#8052=DIRECTION('ref_axis',(1.,0.,0.));
#8053=DIRECTION('',(0.,0.,1.));
#8054=DIRECTION('center_axis',(0.,0.,1.));
#8055=DIRECTION('ref_axis',(1.,0.,0.));
#8056=DIRECTION('center_axis',(0.,0.,1.));
#8057=DIRECTION('ref_axis',(1.,0.,0.));
#8058=DIRECTION('',(0.,0.,-1.));
#8059=DIRECTION('center_axis',(0.,0.,-1.));
#8060=DIRECTION('ref_axis',(1.,0.,0.));
#8061=DIRECTION('',(0.,0.,1.));
#8062=DIRECTION('center_axis',(0.,0.,1.));
#8063=DIRECTION('ref_axis',(1.,0.,0.));
#8064=DIRECTION('',(0.,0.,-1.));
#8065=DIRECTION('center_axis',(0.,0.,-1.));
#8066=DIRECTION('ref_axis',(1.,0.,0.));
#8067=DIRECTION('',(0.,0.,1.));
#8068=DIRECTION('center_axis',(0.,0.,1.));
#8069=DIRECTION('ref_axis',(1.,0.,0.));
#8070=DIRECTION('center_axis',(0.,0.,1.));
#8071=DIRECTION('ref_axis',(1.,0.,0.));
#8072=DIRECTION('center_axis',(0.,0.,1.));
#8073=DIRECTION('ref_axis',(1.,0.,0.));
#8074=DIRECTION('',(0.,0.,1.));
#8075=DIRECTION('center_axis',(0.,0.,1.));
#8076=DIRECTION('ref_axis',(1.,0.,0.));
#8077=DIRECTION('center_axis',(0.,0.,1.));
#8078=DIRECTION('ref_axis',(1.,0.,0.));
#8079=DIRECTION('center_axis',(0.,0.,1.));
#8080=DIRECTION('ref_axis',(1.,0.,0.));
#8081=DIRECTION('',(0.,0.,1.));
#8082=DIRECTION('center_axis',(0.,0.,1.));
#8083=DIRECTION('ref_axis',(1.,0.,0.));
#8084=DIRECTION('center_axis',(0.,0.,1.));
#8085=DIRECTION('ref_axis',(1.,0.,0.));
#8086=DIRECTION('center_axis',(0.,0.,1.));
#8087=DIRECTION('ref_axis',(1.,0.,0.));
#8088=DIRECTION('',(0.,0.,1.));
#8089=DIRECTION('center_axis',(0.,0.,1.));
#8090=DIRECTION('ref_axis',(1.,0.,0.));
#8091=DIRECTION('center_axis',(0.,0.,1.));
#8092=DIRECTION('ref_axis',(1.,0.,0.));
#8093=DIRECTION('',(0.,1.,0.));
#8094=DIRECTION('',(1.,0.,0.));
#8095=DIRECTION('',(1.70803542250024E-16,1.,0.));
#8096=DIRECTION('center_axis',(0.,0.,-1.));
#8097=DIRECTION('ref_axis',(1.,0.,0.));
#8098=DIRECTION('',(-3.41607084500048E-16,-1.,0.));
#8099=DIRECTION('',(1.,0.,0.));
#8100=DIRECTION('',(0.,-1.,0.));
#8101=DIRECTION('center_axis',(0.,0.,1.));
#8102=DIRECTION('ref_axis',(1.,0.,0.));
#8103=DIRECTION('center_axis',(0.,0.,1.));
#8104=DIRECTION('ref_axis',(1.,0.,0.));
#8105=DIRECTION('',(-1.,0.,0.));
#8106=DIRECTION('',(0.,1.,0.));
#8107=DIRECTION('',(-1.,0.,0.));
#8108=DIRECTION('center_axis',(0.,0.,-1.));
#8109=DIRECTION('ref_axis',(1.,0.,0.));
#8110=DIRECTION('',(1.,0.,0.));
#8111=DIRECTION('',(0.,1.,0.));
#8112=DIRECTION('',(1.,0.,0.));
#8113=DIRECTION('center_axis',(0.,0.,1.));
#8114=DIRECTION('ref_axis',(1.,0.,0.));
#8115=DIRECTION('',(0.,-1.,0.));
#8116=DIRECTION('',(-1.,0.,0.));
#8117=DIRECTION('',(0.,-1.,0.));
#8118=DIRECTION('center_axis',(0.,0.,-1.));
#8119=DIRECTION('ref_axis',(1.,0.,0.));
#8120=DIRECTION('',(0.,1.,0.));
#8121=DIRECTION('',(-1.,0.,0.));
#8122=DIRECTION('',(0.,1.,0.));
#8123=DIRECTION('center_axis',(0.,0.,1.));
#8124=DIRECTION('ref_axis',(1.,0.,0.));
#8125=DIRECTION('',(1.,-1.11022302462516E-16,0.));
#8126=DIRECTION('',(0.,-1.,0.));
#8127=DIRECTION('',(1.,-1.06752213906265E-16,0.));
#8128=DIRECTION('center_axis',(0.,0.,-1.));
#8129=DIRECTION('ref_axis',(1.,0.,0.));
#8130=DIRECTION('',(-1.,1.28102656687518E-16,0.));
#8131=DIRECTION('',(0.,-1.,0.));
#8132=DIRECTION('',(-1.,5.55111512312578E-17,0.));
#8133=DIRECTION('center_axis',(0.,0.,1.));
#8134=DIRECTION('ref_axis',(1.,0.,0.));
#8135=DIRECTION('center_axis',(0.,0.,1.));
#8136=DIRECTION('ref_axis',(1.,0.,0.));
#8137=DIRECTION('center_axis',(0.,0.,1.));
#8138=DIRECTION('ref_axis',(1.,0.,0.));
#8139=DIRECTION('',(0.,0.,1.));
#8140=DIRECTION('center_axis',(0.,0.,1.));
#8141=DIRECTION('ref_axis',(1.,0.,0.));
#8142=DIRECTION('',(0.,0.,-1.));
#8143=DIRECTION('center_axis',(0.,0.,1.));
#8144=DIRECTION('ref_axis',(1.,0.,0.));
#8145=DIRECTION('center_axis',(1.,0.,0.));
#8146=DIRECTION('ref_axis',(0.,1.,0.));
#8147=DIRECTION('',(0.,0.,1.));
#8148=DIRECTION('',(0.,1.,0.));
#8149=DIRECTION('center_axis',(0.,1.,0.));
#8150=DIRECTION('ref_axis',(-1.,0.,0.));
#8151=DIRECTION('',(0.,0.,1.));
#8152=DIRECTION('',(-1.,0.,0.));
#8153=DIRECTION('center_axis',(0.,1.,0.));
#8154=DIRECTION('ref_axis',(-1.,0.,0.));
#8155=DIRECTION('',(0.,0.,1.));
#8156=DIRECTION('',(-1.,0.,0.));
#8157=DIRECTION('',(0.,0.,-1.));
#8158=DIRECTION('center_axis',(-1.,0.,0.));
#8159=DIRECTION('ref_axis',(0.,-1.,0.));
#8160=DIRECTION('',(0.,-1.,0.));
#8161=DIRECTION('center_axis',(-1.,1.70803542250024E-16,0.));
#8162=DIRECTION('ref_axis',(-1.70803542250024E-16,-1.,0.));
#8163=DIRECTION('',(-1.70803542250024E-16,-1.,0.));
#8164=DIRECTION('',(0.,0.,1.));
#8165=DIRECTION('center_axis',(0.,0.,1.));
#8166=DIRECTION('ref_axis',(1.,0.,0.));
#8167=DIRECTION('center_axis',(0.,0.,1.));
#8168=DIRECTION('ref_axis',(1.,0.,0.));
#8169=DIRECTION('',(1.,-5.55111512312578E-17,0.));
#8170=DIRECTION('',(0.,1.,0.));
#8171=DIRECTION('',(1.,-1.28102656687518E-16,0.));
#8172=DIRECTION('center_axis',(0.,0.,1.));
#8173=DIRECTION('ref_axis',(1.,0.,0.));
#8174=DIRECTION('center_axis',(0.,0.,1.));
#8175=DIRECTION('ref_axis',(1.,0.,0.));
#8176=DIRECTION('center_axis',(0.,0.,1.));
#8177=DIRECTION('ref_axis',(1.,0.,0.));
#8178=DIRECTION('center_axis',(0.,0.,1.));
#8179=DIRECTION('ref_axis',(1.,0.,0.));
#8180=DIRECTION('',(3.41607084500048E-16,1.,0.));
#8181=DIRECTION('center_axis',(0.,0.,1.));
#8182=DIRECTION('ref_axis',(1.,0.,0.));
#8183=DIRECTION('center_axis',(0.,0.,1.));
#8184=DIRECTION('ref_axis',(1.,0.,0.));
#8185=DIRECTION('center_axis',(0.,0.,1.));
#8186=DIRECTION('ref_axis',(1.,0.,0.));
#8187=DIRECTION('',(1.,0.,0.));
#8188=DIRECTION('',(0.,-1.,0.));
#8189=DIRECTION('',(1.,0.,0.));
#8190=DIRECTION('center_axis',(0.,0.,1.));
#8191=DIRECTION('ref_axis',(1.,0.,0.));
#8192=DIRECTION('center_axis',(0.,0.,-1.));
#8193=DIRECTION('ref_axis',(1.,0.,0.));
#8194=DIRECTION('center_axis',(0.,0.,1.));
#8195=DIRECTION('ref_axis',(1.,0.,0.));
#8196=DIRECTION('center_axis',(0.,0.,1.));
#8197=DIRECTION('ref_axis',(1.,0.,0.));
#8198=DIRECTION('',(0.,0.,-1.));
#8199=DIRECTION('',(0.,0.,1.));
#8200=DIRECTION('',(0.,0.,1.));
#8201=DIRECTION('center_axis',(0.,0.,1.));
#8202=DIRECTION('ref_axis',(1.,0.,0.));
#8203=DIRECTION('',(0.,0.,-1.));
#8204=DIRECTION('center_axis',(0.,0.,-1.));
#8205=DIRECTION('ref_axis',(1.,0.,0.));
#8206=DIRECTION('',(0.,0.,-1.));
#8207=DIRECTION('center_axis',(0.,0.,1.));
#8208=DIRECTION('ref_axis',(1.,0.,0.));
#8209=DIRECTION('center_axis',(0.,0.,-1.));
#8210=DIRECTION('ref_axis',(1.,0.,0.));
#8211=DIRECTION('',(0.,0.,1.));
#8212=DIRECTION('center_axis',(0.,0.,1.));
#8213=DIRECTION('ref_axis',(1.,0.,0.));
#8214=DIRECTION('',(0.,0.,-1.));
#8215=DIRECTION('center_axis',(0.,0.,-1.));
#8216=DIRECTION('ref_axis',(1.,0.,0.));
#8217=DIRECTION('',(0.,0.,1.));
#8218=DIRECTION('center_axis',(0.,0.,1.));
#8219=DIRECTION('ref_axis',(1.,0.,0.));
#8220=DIRECTION('',(0.,0.,-1.));
#8221=DIRECTION('center_axis',(0.,0.,-1.));
#8222=DIRECTION('ref_axis',(1.,0.,0.));
#8223=DIRECTION('',(0.,0.,1.));
#8224=DIRECTION('center_axis',(1.,-3.41607084500048E-16,0.));
#8225=DIRECTION('ref_axis',(3.41607084500048E-16,1.,0.));
#8226=DIRECTION('center_axis',(0.,0.,1.));
#8227=DIRECTION('ref_axis',(1.,0.,0.));
#8228=DIRECTION('',(0.,0.,-1.));
#8229=DIRECTION('center_axis',(-5.55111512312578E-17,-1.,0.));
#8230=DIRECTION('ref_axis',(1.,-5.55111512312578E-17,0.));
#8231=DIRECTION('',(0.,0.,1.));
#8232=DIRECTION('center_axis',(1.,0.,0.));
#8233=DIRECTION('ref_axis',(0.,1.,0.));
#8234=DIRECTION('',(0.,0.,1.));
#8235=DIRECTION('center_axis',(1.,0.,0.));
#8236=DIRECTION('ref_axis',(0.,1.,0.));
#8237=DIRECTION('',(0.,0.,1.));
#8238=DIRECTION('',(0.,1.,0.));
#8239=DIRECTION('',(0.,0.,-1.));
#8240=DIRECTION('center_axis',(1.11022302462516E-16,1.,0.));
#8241=DIRECTION('ref_axis',(-1.,1.11022302462516E-16,0.));
#8242=DIRECTION('',(-1.,1.11022302462516E-16,0.));
#8243=DIRECTION('center_axis',(1.06752213906265E-16,1.,0.));
#8244=DIRECTION('ref_axis',(-1.,1.06752213906265E-16,0.));
#8245=DIRECTION('',(-1.,1.06752213906265E-16,0.));
#8246=DIRECTION('',(0.,0.,1.));
#8247=DIRECTION('center_axis',(0.,0.,1.));
#8248=DIRECTION('ref_axis',(1.,0.,0.));
#8249=DIRECTION('center_axis',(0.,0.,1.));
#8250=DIRECTION('ref_axis',(1.,0.,0.));
#8251=DIRECTION('',(0.,-1.,0.));
#8252=DIRECTION('',(1.,0.,0.));
#8253=DIRECTION('',(0.,-1.,0.));
#8254=DIRECTION('center_axis',(0.,0.,1.));
#8255=DIRECTION('ref_axis',(1.,0.,0.));
#8256=DIRECTION('center_axis',(0.,0.,1.));
#8257=DIRECTION('ref_axis',(1.,0.,0.));
#8258=DIRECTION('center_axis',(0.,0.,1.));
#8259=DIRECTION('ref_axis',(1.,0.,0.));
#8260=DIRECTION('center_axis',(0.,0.,1.));
#8261=DIRECTION('ref_axis',(1.,0.,0.));
#8262=DIRECTION('center_axis',(0.,0.,1.));
#8263=DIRECTION('ref_axis',(1.,0.,0.));
#8264=DIRECTION('',(0.,0.,1.));
#8265=DIRECTION('center_axis',(-1.28102656687518E-16,-1.,0.));
#8266=DIRECTION('ref_axis',(1.,-1.28102656687518E-16,0.));
#8267=DIRECTION('center_axis',(0.,0.,1.));
#8268=DIRECTION('ref_axis',(1.,0.,0.));
#8269=DIRECTION('',(0.,0.,-1.));
#8270=DIRECTION('center_axis',(-1.,0.,0.));
#8271=DIRECTION('ref_axis',(0.,-1.,0.));
#8272=DIRECTION('',(0.,0.,1.));
#8273=DIRECTION('center_axis',(0.,-1.,0.));
#8274=DIRECTION('ref_axis',(1.,0.,0.));
#8275=DIRECTION('',(0.,0.,1.));
#8276=DIRECTION('center_axis',(0.,-1.,0.));
#8277=DIRECTION('ref_axis',(1.,0.,0.));
#8278=DIRECTION('',(0.,0.,1.));
#8279=DIRECTION('',(1.,0.,0.));
#8280=DIRECTION('',(0.,0.,-1.));
#8281=DIRECTION('center_axis',(1.,0.,0.));
#8282=DIRECTION('ref_axis',(0.,1.,0.));
#8283=DIRECTION('',(0.,1.,0.));
#8284=DIRECTION('center_axis',(1.,0.,0.));
#8285=DIRECTION('ref_axis',(0.,1.,0.));
#8286=DIRECTION('',(0.,1.,0.));
#8287=DIRECTION('',(0.,0.,1.));
#8288=DIRECTION('center_axis',(0.,0.,1.));
#8289=DIRECTION('ref_axis',(1.,0.,0.));
#8290=DIRECTION('center_axis',(0.,0.,1.));
#8291=DIRECTION('ref_axis',(1.,0.,0.));
#8292=DIRECTION('',(-1.,0.,0.));
#8293=DIRECTION('',(0.,-1.,0.));
#8294=DIRECTION('',(-1.,0.,0.));
#8295=DIRECTION('center_axis',(0.,0.,1.));
#8296=DIRECTION('ref_axis',(1.,0.,0.));
#8297=DIRECTION('center_axis',(0.,0.,1.));
#8298=DIRECTION('ref_axis',(1.,0.,0.));
#8299=DIRECTION('center_axis',(0.,0.,1.));
#8300=DIRECTION('ref_axis',(1.,0.,0.));
#8301=DIRECTION('center_axis',(0.,0.,1.));
#8302=DIRECTION('ref_axis',(1.,0.,0.));
#8303=DIRECTION('center_axis',(0.,0.,1.));
#8304=DIRECTION('ref_axis',(1.,0.,0.));
#8305=DIRECTION('',(0.,0.,1.));
#8306=DIRECTION('center_axis',(-1.,0.,0.));
#8307=DIRECTION('ref_axis',(0.,-1.,0.));
#8308=DIRECTION('center_axis',(0.,0.,1.));
#8309=DIRECTION('ref_axis',(1.,0.,0.));
#8310=DIRECTION('',(0.,0.,-1.));
#8311=DIRECTION('center_axis',(0.,1.,0.));
#8312=DIRECTION('ref_axis',(-1.,0.,0.));
#8313=DIRECTION('',(0.,0.,1.));
#8314=DIRECTION('center_axis',(0.,-1.,0.));
#8315=DIRECTION('ref_axis',(1.,0.,0.));
#8316=DIRECTION('',(0.,0.,1.));
#8317=DIRECTION('center_axis',(-1.,0.,0.));
#8318=DIRECTION('ref_axis',(0.,-1.,0.));
#8319=DIRECTION('',(0.,0.,-1.));
#8320=DIRECTION('center_axis',(-1.,0.,0.));
#8321=DIRECTION('ref_axis',(0.,-1.,0.));
#8322=DIRECTION('',(0.,0.,1.));
#8323=DIRECTION('center_axis',(0.,0.,1.));
#8324=DIRECTION('ref_axis',(1.,0.,0.));
#8325=DIRECTION('center_axis',(0.,0.,1.));
#8326=DIRECTION('ref_axis',(1.,0.,0.));
#8327=DIRECTION('center_axis',(0.,0.,1.));
#8328=DIRECTION('ref_axis',(-1.,1.22464679914735E-16,0.));
#8329=DIRECTION('',(0.,0.,1.));
#8330=DIRECTION('',(0.,0.,1.));
#8331=DIRECTION('center_axis',(0.,1.,0.));
#8332=DIRECTION('ref_axis',(-1.,0.,0.));
#8333=DIRECTION('center_axis',(0.,-1.,0.));
#8334=DIRECTION('ref_axis',(1.,0.,0.));
#8335=DIRECTION('center_axis',(0.,0.,1.));
#8336=DIRECTION('ref_axis',(1.,0.,0.));
#8337=DIRECTION('center_axis',(0.,0.,-1.));
#8338=DIRECTION('ref_axis',(1.,0.,0.));
#8339=DIRECTION('center_axis',(0.,0.,1.));
#8340=DIRECTION('ref_axis',(1.,0.,0.));
#8341=DIRECTION('',(0.,0.,-1.));
#8342=DIRECTION('center_axis',(0.,0.,1.));
#8343=DIRECTION('ref_axis',(1.,0.,0.));
#8344=DIRECTION('center_axis',(0.,0.,1.));
#8345=DIRECTION('ref_axis',(1.,0.,0.));
#10187=CARTESIAN_POINT('',(0.,0.,0.));
#10188=CARTESIAN_POINT('Origin',(2.9698484809835,-1.27279220613579,5.9));
#10189=CARTESIAN_POINT('',(2.8048484809835,-1.27279220613579,6.));
#10190=CARTESIAN_POINT('Origin',(2.9698484809835,-1.27279220613579,6.));
#10191=CARTESIAN_POINT('',(2.8048484809835,-1.27279220613579,6.8));
#10192=CARTESIAN_POINT('',(2.8048484809835,-1.27279220613579,5.9));
#10193=CARTESIAN_POINT('Origin',(2.9698484809835,-1.27279220613579,6.8));
#10194=CARTESIAN_POINT('Origin',(2.9698484809835,1.27279220613579,5.9));
#10195=CARTESIAN_POINT('',(2.8048484809835,1.27279220613579,6.));
#10196=CARTESIAN_POINT('Origin',(2.9698484809835,1.27279220613579,6.));
#10197=CARTESIAN_POINT('',(2.8048484809835,1.27279220613579,6.8));
#10198=CARTESIAN_POINT('',(2.8048484809835,1.27279220613579,5.9));
#10199=CARTESIAN_POINT('Origin',(2.9698484809835,1.27279220613579,6.8));
#10200=CARTESIAN_POINT('Origin',(5.51543289325507,1.27279220613579,5.9));
#10201=CARTESIAN_POINT('',(5.35043289325507,1.27279220613579,6.));
#10202=CARTESIAN_POINT('Origin',(5.51543289325507,1.27279220613579,6.));
#10203=CARTESIAN_POINT('',(5.35043289325507,1.27279220613579,6.8));
#10204=CARTESIAN_POINT('',(5.35043289325507,1.27279220613579,5.9));
#10205=CARTESIAN_POINT('Origin',(5.51543289325507,1.27279220613579,6.8));
#10206=CARTESIAN_POINT('Origin',(5.51543289325507,-1.27279220613579,5.9));
#10207=CARTESIAN_POINT('',(5.35043289325507,-1.27279220613579,6.));
#10208=CARTESIAN_POINT('Origin',(5.51543289325507,-1.27279220613579,6.));
#10209=CARTESIAN_POINT('',(5.35043289325507,-1.27279220613579,6.8));
#10210=CARTESIAN_POINT('',(5.35043289325507,-1.27279220613579,5.9));
#10211=CARTESIAN_POINT('Origin',(5.51543289325507,-1.27279220613579,6.8));
#10212=CARTESIAN_POINT('Origin',(1.24264068711928,-3.,5.9));
#10213=CARTESIAN_POINT('',(3.04549806673909,-2.75079071295314,6.));
#10214=CARTESIAN_POINT('',(1.49184997416615,-1.19714262038019,6.));
#10215=CARTESIAN_POINT('Origin',(1.24264068711928,-3.,6.));
#10216=CARTESIAN_POINT('',(3.04549806673909,-2.75079071295314,6.8));
#10217=CARTESIAN_POINT('',(3.04549806673909,-2.75079071295314,5.9));
#10218=CARTESIAN_POINT('',(1.49184997416615,-1.19714262038019,6.8));
#10219=CARTESIAN_POINT('Origin',(1.24264068711928,-3.,6.8));
#10220=CARTESIAN_POINT('',(1.49184997416615,-1.19714262038019,5.9));
#10221=CARTESIAN_POINT('Origin',(1.24264068711929,3.,5.9));
#10222=CARTESIAN_POINT('',(1.49184997416615,1.19714262038019,6.));
#10223=CARTESIAN_POINT('',(3.04549806673909,2.75079071295314,6.));
#10224=CARTESIAN_POINT('Origin',(1.24264068711929,3.,6.));
#10225=CARTESIAN_POINT('',(1.49184997416615,1.19714262038019,6.8));
#10226=CARTESIAN_POINT('',(1.49184997416615,1.19714262038019,5.9));
#10227=CARTESIAN_POINT('',(3.04549806673909,2.75079071295314,6.8));
#10228=CARTESIAN_POINT('Origin',(1.24264068711929,3.,6.8));
#10229=CARTESIAN_POINT('',(3.04549806673909,2.75079071295314,5.9));
#10230=CARTESIAN_POINT('Origin',(7.24264068711929,3.,5.9));
#10231=CARTESIAN_POINT('',(5.43978330749948,2.75079071295314,6.));
#10232=CARTESIAN_POINT('',(6.99343140007243,1.19714262038019,6.));
#10233=CARTESIAN_POINT('Origin',(7.24264068711929,3.,6.));
#10234=CARTESIAN_POINT('',(5.43978330749948,2.75079071295314,6.8));
#10235=CARTESIAN_POINT('',(5.43978330749948,2.75079071295314,5.9));
#10236=CARTESIAN_POINT('',(6.99343140007243,1.19714262038019,6.8));
#10237=CARTESIAN_POINT('Origin',(7.24264068711929,3.,6.8));
#10238=CARTESIAN_POINT('',(6.99343140007243,1.19714262038019,5.9));
#10239=CARTESIAN_POINT('Origin',(7.24264068711929,-3.,5.9));
#10240=CARTESIAN_POINT('',(6.99343140007242,-1.19714262038019,6.8));
#10241=CARTESIAN_POINT('',(6.99343140007242,-1.19714262038019,6.));
#10242=CARTESIAN_POINT('',(6.99343140007243,-1.19714262038019,5.9));
#10243=CARTESIAN_POINT('',(5.43978330749948,-2.75079071295314,6.8));
#10244=CARTESIAN_POINT('Origin',(7.24264068711929,-3.,6.8));
#10245=CARTESIAN_POINT('',(5.43978330749948,-2.75079071295314,6.));
#10246=CARTESIAN_POINT('',(5.43978330749948,-2.75079071295314,5.9));
#10247=CARTESIAN_POINT('Origin',(7.24264068711929,-3.,6.));
#10248=CARTESIAN_POINT('Origin',(4.24264068711929,0.,6.));
#10249=CARTESIAN_POINT('',(3.81264068711929,-2.96902340846279,6.));
#10250=CARTESIAN_POINT('Origin',(4.24264068711929,0.,6.));
#10251=CARTESIAN_POINT('',(3.81264068711929,-2.96902340846279,6.8));
#10252=CARTESIAN_POINT('',(3.81264068711929,-2.96902340846279,6.));
#10253=CARTESIAN_POINT('Origin',(4.24264068711929,0.,6.8));
#10254=CARTESIAN_POINT('Origin',(4.24264068711929,0.,6.));
#10255=CARTESIAN_POINT('',(1.2736172786565,0.43,6.));
#10256=CARTESIAN_POINT('Origin',(4.24264068711929,0.,6.));
#10257=CARTESIAN_POINT('',(1.2736172786565,0.43,6.8));
#10258=CARTESIAN_POINT('',(1.2736172786565,0.43,6.));
#10259=CARTESIAN_POINT('Origin',(4.24264068711929,0.,6.8));
#10260=CARTESIAN_POINT('Origin',(4.24264068711929,0.,6.));
#10261=CARTESIAN_POINT('',(4.67264068711929,2.96902340846279,6.));
#10262=CARTESIAN_POINT('Origin',(4.24264068711929,0.,6.));
#10263=CARTESIAN_POINT('',(4.67264068711929,2.96902340846279,6.8));
#10264=CARTESIAN_POINT('',(4.67264068711929,2.96902340846279,6.));
#10265=CARTESIAN_POINT('Origin',(4.24264068711929,0.,6.8));
#10266=CARTESIAN_POINT('Origin',(4.24264068711929,0.,6.8));
#10267=CARTESIAN_POINT('',(3.81264068711929,-2.6,6.8));
#10268=CARTESIAN_POINT('',(3.81264068711929,-1.3,6.8));
#10269=CARTESIAN_POINT('',(3.92264068711928,-2.6,6.8));
#10270=CARTESIAN_POINT('',(4.45764068711929,-2.6,6.8));
#10271=CARTESIAN_POINT('',(3.92264068711928,-1.,6.8));
#10272=CARTESIAN_POINT('',(3.92264068711929,-0.5,6.8));
#10273=CARTESIAN_POINT('',(4.56264068711929,-1.,6.8));
#10274=CARTESIAN_POINT('Origin',(4.24264068711929,-1.,6.8));
#10275=CARTESIAN_POINT('',(4.56264068711929,-2.6,6.8));
#10276=CARTESIAN_POINT('',(4.56264068711929,-1.8,6.8));
#10277=CARTESIAN_POINT('',(4.67264068711928,-2.6,6.8));
#10278=CARTESIAN_POINT('',(4.45764068711929,-2.6,6.8));
#10279=CARTESIAN_POINT('',(4.67264068711928,-2.96902340846279,6.8));
#10280=CARTESIAN_POINT('',(4.67264068711929,-1.8,6.8));
#10281=CARTESIAN_POINT('Origin',(4.24264068711929,0.,6.8));
#10282=CARTESIAN_POINT('',(7.21166409558207,-0.43,6.8));
#10283=CARTESIAN_POINT('Origin',(4.24264068711929,0.,6.8));
#10284=CARTESIAN_POINT('',(6.84264068711929,-0.43,6.8));
#10285=CARTESIAN_POINT('',(5.54264068711929,-0.43,6.8));
#10286=CARTESIAN_POINT('',(6.84264068711929,-0.32,6.8));
#10287=CARTESIAN_POINT('',(6.84264068711929,0.215,6.8));
#10288=CARTESIAN_POINT('',(5.24264068711929,-0.32,6.8));
#10289=CARTESIAN_POINT('',(4.74264068711929,-0.32,6.8));
#10290=CARTESIAN_POINT('',(5.24264068711929,0.32,6.8));
#10291=CARTESIAN_POINT('Origin',(5.24264068711929,0.,6.8));
#10292=CARTESIAN_POINT('',(6.84264068711929,0.32,6.8));
#10293=CARTESIAN_POINT('',(6.04264068711929,0.32,6.8));
#10294=CARTESIAN_POINT('',(6.84264068711929,0.43,6.8));
#10295=CARTESIAN_POINT('',(6.84264068711929,0.215,6.8));
#10296=CARTESIAN_POINT('',(7.21166409558207,0.43,6.8));
#10297=CARTESIAN_POINT('',(6.04264068711929,0.43,6.8));
#10298=CARTESIAN_POINT('Origin',(4.24264068711929,0.,6.8));
#10299=CARTESIAN_POINT('',(4.67264068711929,2.6,6.8));
#10300=CARTESIAN_POINT('',(4.67264068711929,1.3,6.8));
#10301=CARTESIAN_POINT('',(4.56264068711929,2.6,6.8));
#10302=CARTESIAN_POINT('',(4.02764068711929,2.6,6.8));
#10303=CARTESIAN_POINT('',(4.56264068711929,1.,6.8));
#10304=CARTESIAN_POINT('',(4.56264068711929,0.5,6.8));
#10305=CARTESIAN_POINT('',(3.92264068711928,1.,6.8));
#10306=CARTESIAN_POINT('Origin',(4.24264068711929,1.,6.8));
#10307=CARTESIAN_POINT('',(3.92264068711929,2.6,6.8));
#10308=CARTESIAN_POINT('',(3.92264068711929,1.8,6.8));
#10309=CARTESIAN_POINT('',(3.81264068711929,2.6,6.8));
#10310=CARTESIAN_POINT('',(4.02764068711929,2.6,6.8));
#10311=CARTESIAN_POINT('',(3.81264068711929,2.96902340846279,6.8));
#10312=CARTESIAN_POINT('',(3.81264068711929,1.8,6.8));
#10313=CARTESIAN_POINT('Origin',(4.24264068711929,0.,6.8));
#10314=CARTESIAN_POINT('',(1.64264068711929,0.43,6.8));
#10315=CARTESIAN_POINT('',(2.94264068711929,0.43,6.8));
#10316=CARTESIAN_POINT('',(1.64264068711929,0.32,6.8));
#10317=CARTESIAN_POINT('',(1.64264068711929,-0.215,6.8));
#10318=CARTESIAN_POINT('',(3.24264068711929,0.32,6.8));
#10319=CARTESIAN_POINT('',(3.74264068711929,0.32,6.8));
#10320=CARTESIAN_POINT('',(3.24264068711929,-0.32,6.8));
#10321=CARTESIAN_POINT('Origin',(3.24264068711929,1.22464679914735E-16,
6.8));
#10322=CARTESIAN_POINT('',(1.64264068711929,-0.32,6.8));
#10323=CARTESIAN_POINT('',(2.44264068711929,-0.32,6.8));
#10324=CARTESIAN_POINT('',(1.64264068711929,-0.43,6.8));
#10325=CARTESIAN_POINT('',(1.64264068711929,-0.215,6.8));
#10326=CARTESIAN_POINT('',(1.2736172786565,-0.43,6.8));
#10327=CARTESIAN_POINT('',(2.44264068711929,-0.43,6.8));
#10328=CARTESIAN_POINT('Origin',(4.24264068711929,0.,6.8));
#10329=CARTESIAN_POINT('Origin',(4.24264068711929,0.,6.));
#10330=CARTESIAN_POINT('',(7.21166409558207,-0.43,6.));
#10331=CARTESIAN_POINT('Origin',(4.24264068711929,0.,6.));
#10332=CARTESIAN_POINT('',(7.21166409558207,-0.43,6.));
#10333=CARTESIAN_POINT('Origin',(4.24264068711929,0.,6.));
#10334=CARTESIAN_POINT('',(4.67264068711928,-2.96902340846279,6.));
#10335=CARTESIAN_POINT('',(4.67264068711928,-2.96902340846279,6.));
#10336=CARTESIAN_POINT('Origin',(4.24264068711929,0.,6.));
#10337=CARTESIAN_POINT('Origin',(4.67264068711928,-3.6,5.9));
#10338=CARTESIAN_POINT('',(4.67264068711928,-2.6,6.));
#10339=CARTESIAN_POINT('',(4.67264068711928,-2.6,5.9));
#10340=CARTESIAN_POINT('',(4.67264068711929,-1.8,6.));
#10341=CARTESIAN_POINT('Origin',(4.67264068711928,-2.6,5.9));
#10342=CARTESIAN_POINT('',(4.56264068711929,-2.6,6.));
#10343=CARTESIAN_POINT('',(4.56264068711929,-2.6,5.9));
#10344=CARTESIAN_POINT('',(4.45764068711929,-2.6,6.));
#10345=CARTESIAN_POINT('Origin',(4.67264068711928,-2.6,5.9));
#10346=CARTESIAN_POINT('',(3.81264068711929,-2.6,6.));
#10347=CARTESIAN_POINT('',(3.81264068711929,-2.6,5.9));
#10348=CARTESIAN_POINT('',(3.92264068711928,-2.6,6.));
#10349=CARTESIAN_POINT('',(4.45764068711929,-2.6,6.));
#10350=CARTESIAN_POINT('',(3.92264068711928,-2.6,5.9));
#10351=CARTESIAN_POINT('Origin',(3.81264068711929,-2.6,5.9));
#10352=CARTESIAN_POINT('',(3.81264068711929,-1.3,6.));
#10353=CARTESIAN_POINT('Origin',(3.92264068711928,-1.,5.9));
#10354=CARTESIAN_POINT('',(3.92264068711928,-1.,6.));
#10355=CARTESIAN_POINT('',(3.92264068711929,-0.5,6.));
#10356=CARTESIAN_POINT('',(3.92264068711928,-1.,5.9));
#10357=CARTESIAN_POINT('Origin',(4.24264068711929,0.,6.));
#10358=CARTESIAN_POINT('',(1.2736172786565,-0.43,6.));
#10359=CARTESIAN_POINT('Origin',(4.24264068711929,0.,6.));
#10360=CARTESIAN_POINT('',(1.64264068711929,-0.43,6.));
#10361=CARTESIAN_POINT('',(2.44264068711929,-0.43,6.));
#10362=CARTESIAN_POINT('',(1.64264068711929,-0.32,6.));
#10363=CARTESIAN_POINT('',(1.64264068711929,-0.215,6.));
#10364=CARTESIAN_POINT('',(3.24264068711929,-0.32,6.));
#10365=CARTESIAN_POINT('',(2.44264068711929,-0.32,6.));
#10366=CARTESIAN_POINT('',(3.54884068711929,-0.0929599913941466,6.));
#10367=CARTESIAN_POINT('Origin',(3.24264068711929,1.22464679914735E-16,
6.));
#10368=CARTESIAN_POINT('',(4.14968069572514,-0.6938,6.));
#10369=CARTESIAN_POINT('Origin',(4.24264068711929,0.,6.));
#10370=CARTESIAN_POINT('Origin',(4.24264068711929,-1.,6.));
#10371=CARTESIAN_POINT('Origin',(4.24264068711929,0.,6.));
#10372=CARTESIAN_POINT('',(4.56264068711929,-1.,6.));
#10373=CARTESIAN_POINT('',(4.56264068711929,-1.8,6.));
#10374=CARTESIAN_POINT('',(4.33560067851344,-0.6938,6.));
#10375=CARTESIAN_POINT('Origin',(4.24264068711929,-1.,6.));
#10376=CARTESIAN_POINT('',(4.93644068711929,-0.0929599913941494,6.));
#10377=CARTESIAN_POINT('Origin',(4.24264068711929,0.,6.));
#10378=CARTESIAN_POINT('',(5.24264068711929,-0.32,6.));
#10379=CARTESIAN_POINT('Origin',(5.24264068711929,0.,6.));
#10380=CARTESIAN_POINT('',(6.84264068711929,-0.32,6.));
#10381=CARTESIAN_POINT('',(4.74264068711929,-0.32,6.));
#10382=CARTESIAN_POINT('',(6.84264068711929,-0.43,6.));
#10383=CARTESIAN_POINT('',(6.84264068711929,0.215,6.));
#10384=CARTESIAN_POINT('',(5.54264068711929,-0.43,6.));
#10385=CARTESIAN_POINT('Origin',(4.24264068711929,-1.,5.9));
#10386=CARTESIAN_POINT('',(4.33560067851343,-0.6938,5.9));
#10387=CARTESIAN_POINT('',(4.14968069572514,-0.6938,5.9));
#10388=CARTESIAN_POINT('Origin',(4.24264068711929,0.,5.9));
#10389=CARTESIAN_POINT('Origin',(4.24264068711929,-1.,5.9));
#10390=CARTESIAN_POINT('Origin',(4.24264068711929,-1.,5.9));
#10391=CARTESIAN_POINT('',(4.33560067851343,-0.6938,5.9));
#10392=CARTESIAN_POINT('',(4.56264068711929,-1.,5.9));
#10393=CARTESIAN_POINT('',(4.14968069572514,-0.6938,5.9));
#10394=CARTESIAN_POINT('Origin',(4.24264068711929,0.,2.95));
#10395=CARTESIAN_POINT('',(3.54884068711929,-0.0929599913941465,5.9));
#10396=CARTESIAN_POINT('',(3.54884068711929,-0.0929599913941465,5.9));
#10397=CARTESIAN_POINT('',(3.54264068711929,-8.57252759403147E-17,5.9));
#10398=CARTESIAN_POINT('Origin',(4.24264068711929,0.,5.9));
#10399=CARTESIAN_POINT('',(3.54264068711929,-8.57252759403147E-17,2.95));
#10400=CARTESIAN_POINT('',(3.54264068711929,-8.57252759403147E-17,2.95));
#10401=CARTESIAN_POINT('Origin',(4.24264068711929,0.,2.95));
#10402=CARTESIAN_POINT('',(3.54884068711929,0.0929599913941467,5.9));
#10403=CARTESIAN_POINT('Origin',(4.24264068711929,0.,5.9));
#10404=CARTESIAN_POINT('',(3.54884068711929,0.0929599913941468,6.));
#10405=CARTESIAN_POINT('',(3.54884068711929,0.0929599913941467,5.9));
#10406=CARTESIAN_POINT('',(4.14968069572514,0.6938,6.));
#10407=CARTESIAN_POINT('Origin',(4.24264068711929,0.,6.));
#10408=CARTESIAN_POINT('',(4.14968069572514,0.6938,5.9));
#10409=CARTESIAN_POINT('',(4.14968069572514,0.6938,5.9));
#10410=CARTESIAN_POINT('',(4.33560067851343,0.6938,5.9));
#10411=CARTESIAN_POINT('Origin',(4.24264068711929,0.,5.9));
#10412=CARTESIAN_POINT('',(4.33560067851344,0.6938,6.));
#10413=CARTESIAN_POINT('',(4.33560067851343,0.6938,5.9));
#10414=CARTESIAN_POINT('',(4.93644068711929,0.0929599913941494,6.));
#10415=CARTESIAN_POINT('Origin',(4.24264068711929,0.,6.));
#10416=CARTESIAN_POINT('',(4.93644068711929,0.0929599913941487,5.9));
#10417=CARTESIAN_POINT('',(4.93644068711929,0.0929599913941487,5.9));
#10418=CARTESIAN_POINT('',(4.93644068711929,-0.0929599913941487,5.9));
#10419=CARTESIAN_POINT('Origin',(4.24264068711929,0.,5.9));
#10420=CARTESIAN_POINT('',(4.93644068711929,-0.0929599913941487,5.9));
#10421=CARTESIAN_POINT('Origin',(4.56264068711929,-3.6,5.9));
#10422=CARTESIAN_POINT('Origin',(4.24264068711929,0.,6.));
#10423=CARTESIAN_POINT('',(1.2736172786565,-0.43,6.));
#10424=CARTESIAN_POINT('Origin',(0.642640687119285,-0.43,5.9));
#10425=CARTESIAN_POINT('',(1.64264068711929,-0.43,5.9));
#10426=CARTESIAN_POINT('Origin',(1.64264068711929,-0.43,5.9));
#10427=CARTESIAN_POINT('',(1.64264068711929,-0.32,5.9));
#10428=CARTESIAN_POINT('Origin',(1.64264068711929,-0.43,5.9));
#10429=CARTESIAN_POINT('',(1.64264068711929,0.43,6.));
#10430=CARTESIAN_POINT('',(1.64264068711929,0.43,5.9));
#10431=CARTESIAN_POINT('',(1.64264068711929,0.32,6.));
#10432=CARTESIAN_POINT('',(1.64264068711929,-0.215,6.));
#10433=CARTESIAN_POINT('',(1.64264068711929,0.32,5.9));
#10434=CARTESIAN_POINT('Origin',(1.64264068711929,0.43,5.9));
#10435=CARTESIAN_POINT('',(2.94264068711929,0.43,6.));
#10436=CARTESIAN_POINT('Origin',(3.24264068711929,0.32,5.9));
#10437=CARTESIAN_POINT('',(3.24264068711929,0.32,6.));
#10438=CARTESIAN_POINT('',(3.74264068711929,0.32,6.));
#10439=CARTESIAN_POINT('',(3.24264068711929,0.32,5.9));
#10440=CARTESIAN_POINT('Origin',(4.24264068711929,0.,6.));
#10441=CARTESIAN_POINT('',(3.81264068711929,2.96902340846279,6.));
#10442=CARTESIAN_POINT('Origin',(4.24264068711929,0.,6.));
#10443=CARTESIAN_POINT('',(3.81264068711929,2.6,6.));
#10444=CARTESIAN_POINT('',(3.81264068711929,1.8,6.));
#10445=CARTESIAN_POINT('',(3.92264068711929,2.6,6.));
#10446=CARTESIAN_POINT('',(4.02764068711929,2.6,6.));
#10447=CARTESIAN_POINT('',(3.92264068711928,1.,6.));
#10448=CARTESIAN_POINT('',(3.92264068711929,1.8,6.));
#10449=CARTESIAN_POINT('Origin',(4.24264068711929,1.,6.));
#10450=CARTESIAN_POINT('Origin',(3.24264068711929,1.22464679914735E-16,
6.));
#10451=CARTESIAN_POINT('Origin',(3.24264068711929,1.11022302462516E-16,
5.9));
#10452=CARTESIAN_POINT('Origin',(3.24264068711929,1.22464679914735E-16,
5.9));
#10453=CARTESIAN_POINT('Origin',(3.24264068711929,1.22464679914735E-16,
5.9));
#10454=CARTESIAN_POINT('',(3.24264068711929,-0.32,5.9));
#10455=CARTESIAN_POINT('Origin',(0.642640687119285,-0.32,5.9));
#10456=CARTESIAN_POINT('Origin',(4.24264068711929,0.,6.));
#10457=CARTESIAN_POINT('',(3.81264068711929,2.96902340846279,6.));
#10458=CARTESIAN_POINT('Origin',(3.81264068711929,3.6,5.9));
#10459=CARTESIAN_POINT('',(3.81264068711929,2.6,5.9));
#10460=CARTESIAN_POINT('Origin',(3.81264068711929,2.6,5.9));
#10461=CARTESIAN_POINT('',(3.92264068711928,2.6,5.9));
#10462=CARTESIAN_POINT('Origin',(3.81264068711929,2.6,5.9));
#10463=CARTESIAN_POINT('',(4.67264068711929,2.6,6.));
#10464=CARTESIAN_POINT('',(4.67264068711929,2.6,5.9));
#10465=CARTESIAN_POINT('',(4.56264068711929,2.6,6.));
#10466=CARTESIAN_POINT('',(4.02764068711929,2.6,6.));
#10467=CARTESIAN_POINT('',(4.56264068711929,2.6,5.9));
#10468=CARTESIAN_POINT('Origin',(4.67264068711929,2.6,5.9));
#10469=CARTESIAN_POINT('',(4.67264068711929,1.3,6.));
#10470=CARTESIAN_POINT('Origin',(4.56264068711929,1.,5.9));
#10471=CARTESIAN_POINT('',(4.56264068711929,1.,6.));
#10472=CARTESIAN_POINT('',(4.56264068711929,0.5,6.));
#10473=CARTESIAN_POINT('',(4.56264068711929,1.,5.9));
#10474=CARTESIAN_POINT('Origin',(4.24264068711929,0.,6.));
#10475=CARTESIAN_POINT('',(7.21166409558207,0.43,6.));
#10476=CARTESIAN_POINT('Origin',(4.24264068711929,0.,6.));
#10477=CARTESIAN_POINT('',(6.84264068711929,0.43,6.));
#10478=CARTESIAN_POINT('',(6.04264068711929,0.43,6.));
#10479=CARTESIAN_POINT('',(6.84264068711929,0.32,6.));
#10480=CARTESIAN_POINT('',(6.84264068711929,0.215,6.));
#10481=CARTESIAN_POINT('',(5.24264068711929,0.32,6.));
#10482=CARTESIAN_POINT('',(6.04264068711929,0.32,6.));
#10483=CARTESIAN_POINT('Origin',(5.24264068711929,0.,6.));
#10484=CARTESIAN_POINT('Origin',(4.24264068711929,1.,6.));
#10485=CARTESIAN_POINT('Origin',(4.24264068711929,1.,5.9));
#10486=CARTESIAN_POINT('Origin',(4.24264068711929,1.,5.9));
#10487=CARTESIAN_POINT('Origin',(4.24264068711929,1.,5.9));
#10488=CARTESIAN_POINT('',(3.92264068711928,1.,5.9));
#10489=CARTESIAN_POINT('Origin',(3.92264068711928,3.6,5.9));
#10490=CARTESIAN_POINT('Origin',(4.24264068711929,0.,6.));
#10491=CARTESIAN_POINT('',(7.21166409558207,0.43,6.));
#10492=CARTESIAN_POINT('Origin',(7.84264068711929,0.43,5.9));
#10493=CARTESIAN_POINT('',(6.84264068711929,0.43,5.9));
#10494=CARTESIAN_POINT('Origin',(6.84264068711929,-0.43,5.9));
#10495=CARTESIAN_POINT('',(6.84264068711929,-0.43,5.9));
#10496=CARTESIAN_POINT('Origin',(6.84264068711929,0.43,5.9));
#10497=CARTESIAN_POINT('',(6.84264068711929,-0.32,5.9));
#10498=CARTESIAN_POINT('Origin',(6.84264068711929,0.43,5.9));
#10499=CARTESIAN_POINT('',(6.84264068711929,0.32,5.9));
#10500=CARTESIAN_POINT('Origin',(5.24264068711929,0.,5.9));
#10501=CARTESIAN_POINT('Origin',(5.24264068711929,0.,5.9));
#10502=CARTESIAN_POINT('Origin',(5.24264068711929,0.,5.9));
#10503=CARTESIAN_POINT('',(5.24264068711929,0.32,5.9));
#10504=CARTESIAN_POINT('',(5.24264068711929,-0.32,5.9));
#10505=CARTESIAN_POINT('Origin',(7.84264068711929,0.32,5.9));
#10506=CARTESIAN_POINT('Origin',(5.24264068711929,-0.32,5.9));
#10507=CARTESIAN_POINT('Origin',(4.24264068711929,0.,2.95));
#10508=CARTESIAN_POINT('',(3.74264068711929,6.12323399573677E-17,2.95));
#10509=CARTESIAN_POINT('Origin',(4.24264068711929,0.,2.95));
#10510=CARTESIAN_POINT('Origin',(4.24264068711929,0.,1.));
#10511=CARTESIAN_POINT('',(3.74264068711929,-6.12323399573677E-17,1.));
#10512=CARTESIAN_POINT('',(3.74264068711929,-6.12323399573677E-17,1.));
#10513=CARTESIAN_POINT('Origin',(4.24264068711929,0.,1.));
#10514=CARTESIAN_POINT('Origin',(4.24264068711929,0.,1.));
#10803=UNCERTAINTY_MEASURE_WITH_UNIT(LENGTH_MEASURE(0.001),#10838,
'DISTANCE_ACCURACY_VALUE',
'Maximum model space distance between geometric entities at asserted c
onnectivities');
#10807=UNCERTAINTY_MEASURE_WITH_UNIT(LENGTH_MEASURE(0.001),#10838,
'DISTANCE_ACCURACY_VALUE',
'Maximum model space distance between geometric entities at asserted c
onnectivities');
#10833=(
GEOMETRIC_REPRESENTATION_CONTEXT(3)
GLOBAL_UNCERTAINTY_ASSIGNED_CONTEXT((#10803))
GLOBAL_UNIT_ASSIGNED_CONTEXT((#10838,#10840,#10841))
REPRESENTATION_CONTEXT('','3D')
);
#10837=(
GEOMETRIC_REPRESENTATION_CONTEXT(3)
GLOBAL_UNCERTAINTY_ASSIGNED_CONTEXT((#10807))
GLOBAL_UNIT_ASSIGNED_CONTEXT((#10838,#10840,#10841))
REPRESENTATION_CONTEXT('','3D')
);
#10838=(
LENGTH_UNIT()
NAMED_UNIT(*)
SI_UNIT(.CENTI.,.METRE.)
);
#10840=(
NAMED_UNIT(*)
PLANE_ANGLE_UNIT()
SI_UNIT($,.RADIAN.)
);
#10841=(
NAMED_UNIT(*)
SI_UNIT($,.STERADIAN.)
SOLID_ANGLE_UNIT()
);
#10867=SHAPE_DEFINITION_REPRESENTATION(#10920,#10966);
#10920=PRODUCT_DEFINITION_SHAPE('',$,#10996);
#10966=SHAPE_REPRESENTATION('',(#6487),#10833);
#10970=PRODUCT_DEFINITION_CONTEXT('part definition',#11059,'design');
#10996=PRODUCT_DEFINITION('Output wheel and spindle',
'Output wheel and spindle',#11025,#10970);
#11025=PRODUCT_DEFINITION_FORMATION('',$,#11086);
#11059=APPLICATION_CONTEXT(
'Core Data for Automotive Mechanical Design Process');
#11060=PRODUCT_CONTEXT('part definition',#11059,'mechanical');
#11086=PRODUCT('Output wheel and spindle','Output wheel and spindle',
'Output wheel and spindle',(#11060));
#11153=COLOUR_RGB('Sky Blue',0.24,0.69,0.87);
#11154=FILL_AREA_STYLE_COLOUR('',#11153);
#11155=FILL_AREA_STYLE('',(#11154));
#11156=SURFACE_STYLE_FILL_AREA(#11155);
#11157=SURFACE_SIDE_STYLE('',(#11156));
#11158=SURFACE_STYLE_USAGE(.BOTH.,#11157);
#11159=PRESENTATION_STYLE_ASSIGNMENT((#11158));
ENDSEC;
END-ISO-10303-21;
